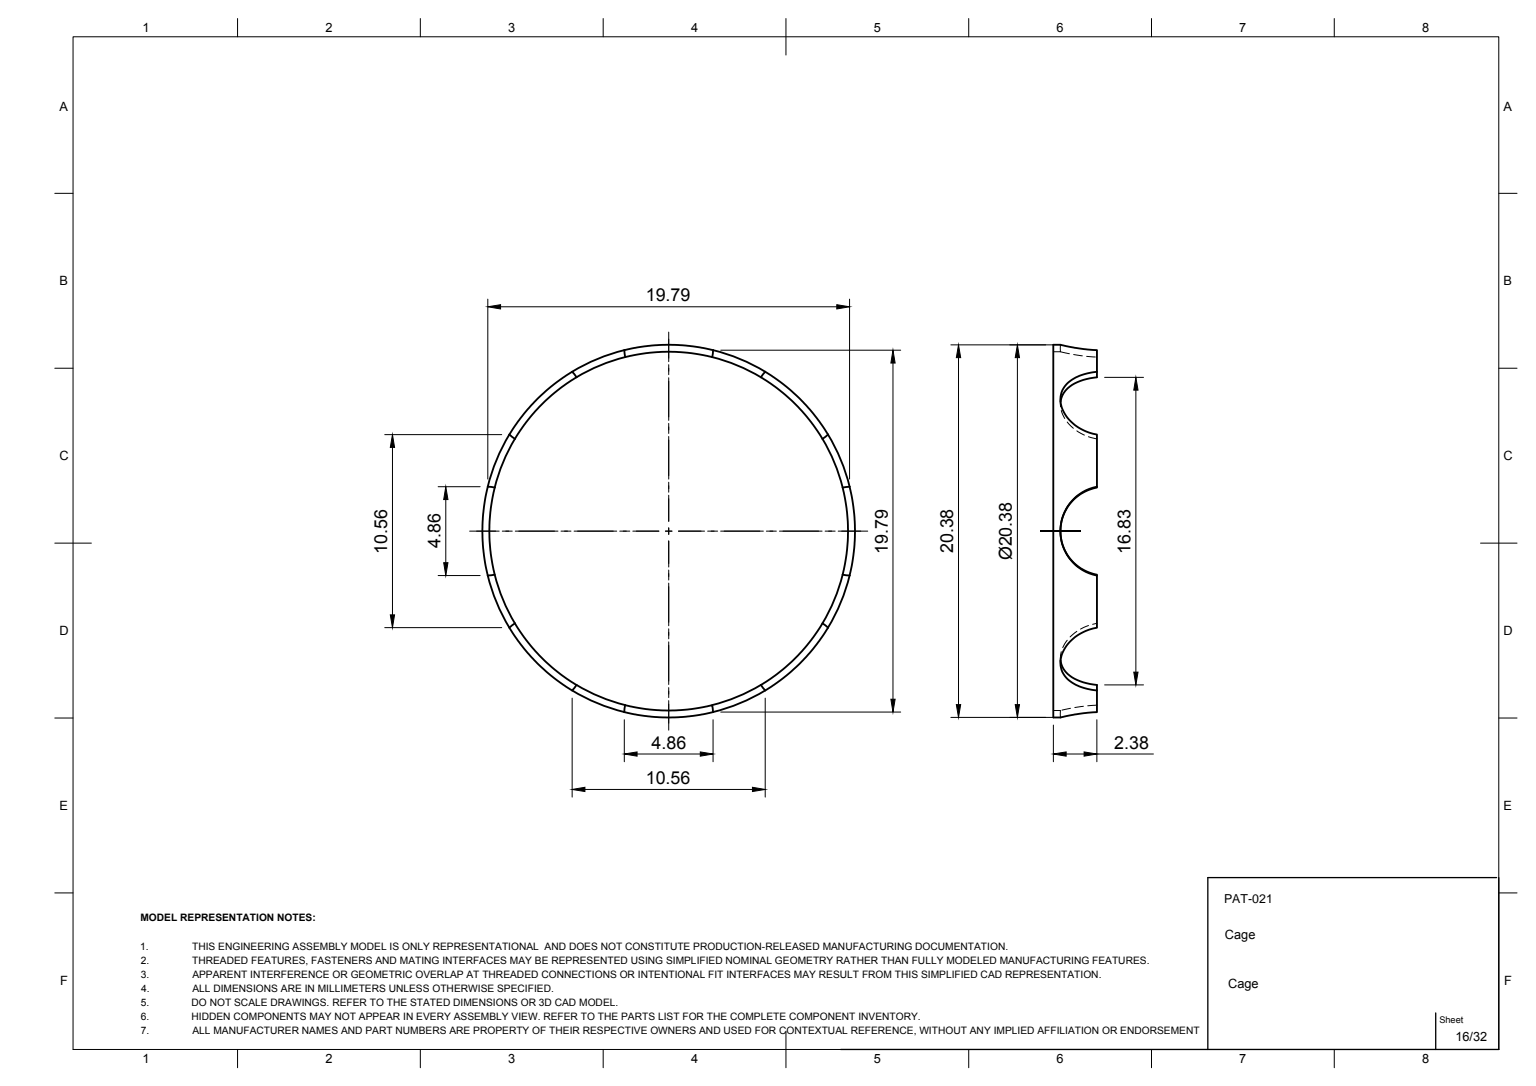
ISO-10303-21;
HEADER;
/* Generated by software containing ST-Developer
 * from STEP Tools, Inc. (www.steptools.com) 
 */

FILE_DESCRIPTION(
/* description */ ('Chain-less indexing wheel (Geneva) drive'),
/* implementation_level */ '2;1');

FILE_NAME(
/* name */ 'Cage.step',
/* time_stamp */ '2026-10-28T03:25:22-07:00',
/* author */ (''),
/* organization */ (''),
/* preprocessor_version */ 'ST-DEVELOPER v20.2',
/* originating_system */ 'Autodesk Translation Framework v15.17.0.0',
/* authorisation */ '');

FILE_SCHEMA (('AUTOMOTIVE_DESIGN { 1 0 10303 214 3 1 1 }'));
ENDSEC;

DATA;
#10=MECHANICAL_DESIGN_GEOMETRIC_PRESENTATION_REPRESENTATION('',(#320),#10957);
#187=SPHERICAL_SURFACE('',#6329,0.247676);
#188=SPHERICAL_SURFACE('',#6345,0.247676);
#189=SPHERICAL_SURFACE('',#6350,0.247676);
#190=SPHERICAL_SURFACE('',#6355,0.247676);
#191=SPHERICAL_SURFACE('',#6360,0.247676);
#192=SPHERICAL_SURFACE('',#6365,0.247676);
#193=SPHERICAL_SURFACE('',#6370,0.247676);
#194=SPHERICAL_SURFACE('',#6378,0.247676);
#215=B_SPLINE_CURVE_WITH_KNOTS('',3,(#9357,#9358,#9359,#9360,#9361,#9362,
#9363,#9364,#9365,#9366,#9367,#9368,#9369,#9370,#9371,#9372,#9373,#9374,
#9375,#9376,#9377,#9378),.UNSPECIFIED.,.F.,.F.,(4,2,2,2,2,2,2,2,2,2,4),
(0.0473477652366656,0.126350602536658,0.189525903804987,0.252701205073317,
0.313298422430275,0.373895639787233,0.434492857144191,0.495090074501149,
0.558265375769478,0.621440677037807,0.7004435143378),.UNSPECIFIED.);
#216=B_SPLINE_CURVE_WITH_KNOTS('',3,(#9382,#9383,#9384,#9385,#9386,#9387,
#9388,#9389,#9390,#9391,#9392,#9393,#9394,#9395,#9396,#9397,#9398,#9399,
#9400,#9401,#9402,#9403),.UNSPECIFIED.,.F.,.F.,(4,2,2,2,2,2,2,2,2,2,4),
(0.0464897534940957,0.0852567806515119,0.170513561303024,0.246687263103517,
0.308657850341199,0.370628437578881,0.432599024816563,0.494569612054245,
0.570743313854739,0.656000094506251,0.694767121663666),.UNSPECIFIED.);
#217=B_SPLINE_CURVE_WITH_KNOTS('',3,(#9409,#9410,#9411,#9412,#9413,#9414,
#9415,#9416,#9417,#9418,#9419,#9420,#9421,#9422,#9423,#9424,#9425,#9426,
#9427,#9428,#9429,#9430),.UNSPECIFIED.,.F.,.F.,(4,2,2,2,2,2,2,2,2,2,4),
(0.0464897534940957,0.0852567806515118,0.170513561303024,0.246687263103517,
0.308657850341199,0.370628437578881,0.432599024816563,0.494569612054245,
0.570743313854738,0.65600009450625,0.694767121663666),.UNSPECIFIED.);
#218=B_SPLINE_CURVE_WITH_KNOTS('',3,(#9434,#9435,#9436,#9437,#9438,#9439,
#9440,#9441,#9442,#9443,#9444,#9445,#9446,#9447,#9448,#9449,#9450,#9451,
#9452,#9453,#9454,#9455),.UNSPECIFIED.,.F.,.F.,(4,2,2,2,2,2,2,2,2,2,4),
(0.0464897534940957,0.0852567806515119,0.170513561303024,0.246687263103517,
0.308657850341199,0.370628437578881,0.432599024816563,0.494569612054245,
0.570743313854739,0.656000094506251,0.694767121663666),.UNSPECIFIED.);
#219=B_SPLINE_CURVE_WITH_KNOTS('',3,(#9459,#9460,#9461,#9462,#9463,#9464,
#9465,#9466,#9467,#9468,#9469,#9470),.UNSPECIFIED.,.F.,.F.,(4,2,2,2,2,4),
(0.0464897534940957,0.0852567806515119,0.170513561303024,0.246687263103517,
0.308657850341199,0.370628437578881),.UNSPECIFIED.);
#220=B_SPLINE_CURVE_WITH_KNOTS('',3,(#9475,#9476,#9477,#9478,#9479,#9480,
#9481,#9482,#9483,#9484,#9485,#9486),.UNSPECIFIED.,.F.,.F.,(4,2,2,2,2,4),
(0.370628437578881,0.432599024816563,0.494569612054245,0.570743313854738,
0.65600009450625,0.694767121663666),.UNSPECIFIED.);
#221=B_SPLINE_CURVE_WITH_KNOTS('',3,(#9490,#9491,#9492,#9493,#9494,#9495,
#9496,#9497,#9498,#9499,#9500,#9501,#9502,#9503,#9504,#9505,#9506,#9507,
#9508,#9509,#9510,#9511),.UNSPECIFIED.,.F.,.F.,(4,2,2,2,2,2,2,2,2,2,4),
(0.0464897534940957,0.0852567806515121,0.170513561303024,0.246687263103518,
0.308657850341199,0.370628437578881,0.432599024816563,0.494569612054245,
0.570743313854738,0.65600009450625,0.694767121663666),.UNSPECIFIED.);
#222=B_SPLINE_CURVE_WITH_KNOTS('',3,(#9515,#9516,#9517,#9518,#9519,#9520,
#9521,#9522,#9523,#9524,#9525,#9526,#9527,#9528,#9529,#9530,#9531,#9532,
#9533,#9534,#9535,#9536),.UNSPECIFIED.,.F.,.F.,(4,2,2,2,2,2,2,2,2,2,4),
(0.0464897534940957,0.0852567806515119,0.170513561303024,0.246687263103517,
0.308657850341199,0.370628437578881,0.432599024816563,0.494569612054245,
0.570743313854738,0.65600009450625,0.694767121663667),.UNSPECIFIED.);
#223=B_SPLINE_CURVE_WITH_KNOTS('',3,(#9540,#9541,#9542,#9543,#9544,#9545,
#9546,#9547,#9548,#9549,#9550,#9551,#9552,#9553,#9554,#9555,#9556,#9557,
#9558,#9559,#9560,#9561),.UNSPECIFIED.,.F.,.F.,(4,2,2,2,2,2,2,2,2,2,4),
(0.0464897534940957,0.0852567806515119,0.170513561303024,0.246687263103517,
0.308657850341199,0.370628437578881,0.432599024816563,0.494569612054245,
0.570743313854738,0.65600009450625,0.694767121663666),.UNSPECIFIED.);
#224=B_SPLINE_CURVE_WITH_KNOTS('',3,(#9565,#9566,#9567,#9568,#9569,#9570,
#9571,#9572,#9573,#9574,#9575,#9576,#9577,#9578,#9579,#9580,#9581,#9582,
#9583,#9584,#9585,#9586),.UNSPECIFIED.,.F.,.F.,(4,2,2,2,2,2,2,2,2,2,4),
(0.0464897534940957,0.0852567806515119,0.170513561303024,0.246687263103517,
0.308657850341199,0.370628437578881,0.432599024816563,0.494569612054245,
0.570743313854739,0.656000094506251,0.694767121663667),.UNSPECIFIED.);
#225=B_SPLINE_CURVE_WITH_KNOTS('',3,(#9594,#9595,#9596,#9597,#9598,#9599,
#9600,#9601,#9602,#9603,#9604,#9605,#9606,#9607,#9608,#9609,#9610,#9611,
#9612,#9613,#9614,#9615),.UNSPECIFIED.,.F.,.F.,(4,2,2,2,2,2,2,2,2,2,4),
(0.0473477652366656,0.126350602536658,0.189525903804987,0.252701205073316,
0.313298422430274,0.373895639787232,0.434492857144191,0.495090074501149,
0.558265375769478,0.621440677037807,0.7004435143378),.UNSPECIFIED.);
#226=B_SPLINE_CURVE_WITH_KNOTS('',3,(#9623,#9624,#9625,#9626,#9627,#9628,
#9629,#9630,#9631,#9632,#9633,#9634,#9635,#9636,#9637,#9638,#9639,#9640,
#9641,#9642,#9643,#9644),.UNSPECIFIED.,.F.,.F.,(4,2,2,2,2,2,2,2,2,2,4),
(0.0473477652366656,0.126350602536658,0.189525903804987,0.252701205073317,
0.313298422430275,0.373895639787233,0.434492857144191,0.495090074501149,
0.558265375769478,0.621440677037807,0.7004435143378),.UNSPECIFIED.);
#227=B_SPLINE_CURVE_WITH_KNOTS('',3,(#9653,#9654,#9655,#9656,#9657,#9658,
#9659,#9660,#9661,#9662,#9663,#9664),.UNSPECIFIED.,.F.,.F.,(4,2,2,2,2,4),
(0.0473477652366656,0.126350602536658,0.189525903804987,0.252701205073316,
0.313298422430275,0.373895639787233),.UNSPECIFIED.);
#228=B_SPLINE_CURVE_WITH_KNOTS('',3,(#9666,#9667,#9668,#9669,#9670,#9671,
#9672,#9673,#9674,#9675,#9676,#9677),.UNSPECIFIED.,.F.,.F.,(4,2,2,2,2,4),
(0.373895639787233,0.434492857144191,0.495090074501149,0.558265375769478,
0.621440677037807,0.7004435143378),.UNSPECIFIED.);
#229=B_SPLINE_CURVE_WITH_KNOTS('',3,(#9684,#9685,#9686,#9687,#9688,#9689,
#9690,#9691,#9692,#9693,#9694,#9695,#9696,#9697,#9698,#9699,#9700,#9701,
#9702,#9703,#9704,#9705),.UNSPECIFIED.,.F.,.F.,(4,2,2,2,2,2,2,2,2,2,4),
(0.0473477652366656,0.126350602536658,0.189525903804987,0.252701205073316,
0.313298422430275,0.373895639787233,0.434492857144191,0.495090074501149,
0.558265375769478,0.621440677037807,0.7004435143378),.UNSPECIFIED.);
#230=B_SPLINE_CURVE_WITH_KNOTS('',3,(#9713,#9714,#9715,#9716,#9717,#9718,
#9719,#9720,#9721,#9722,#9723,#9724,#9725,#9726,#9727,#9728,#9729,#9730,
#9731,#9732,#9733,#9734),.UNSPECIFIED.,.F.,.F.,(4,2,2,2,2,2,2,2,2,2,4),
(0.0473477652366656,0.126350602536658,0.189525903804987,0.252701205073317,
0.313298422430275,0.373895639787233,0.434492857144191,0.495090074501149,
0.558265375769478,0.621440677037807,0.7004435143378),.UNSPECIFIED.);
#231=B_SPLINE_CURVE_WITH_KNOTS('',3,(#9742,#9743,#9744,#9745,#9746,#9747,
#9748,#9749,#9750,#9751,#9752,#9753,#9754,#9755,#9756,#9757,#9758,#9759,
#9760,#9761,#9762,#9763),.UNSPECIFIED.,.F.,.F.,(4,2,2,2,2,2,2,2,2,2,4),
(0.0473477652366656,0.126350602536658,0.189525903804987,0.252701205073316,
0.313298422430275,0.373895639787233,0.434492857144191,0.495090074501149,
0.558265375769478,0.621440677037807,0.7004435143378),.UNSPECIFIED.);
#232=B_SPLINE_CURVE_WITH_KNOTS('',3,(#9772,#9773,#9774,#9775,#9776,#9777,
#9778,#9779,#9780,#9781,#9782,#9783,#9784,#9785,#9786,#9787,#9788,#9789,
#9790,#9791,#9792,#9793),.UNSPECIFIED.,.F.,.F.,(4,2,2,2,2,2,2,2,2,2,4),
(0.0473477652366656,0.126350602536658,0.189525903804987,0.252701205073317,
0.313298422430275,0.373895639787233,0.434492857144191,0.495090074501149,
0.558265375769478,0.621440677037807,0.7004435143378),.UNSPECIFIED.);
#263=SHAPE_REPRESENTATION_RELATIONSHIP('SRR','None',#11077,#288);
#288=ADVANCED_BREP_SHAPE_REPRESENTATION('',(#352),#10940);
#320=STYLED_ITEM('',(#11287),#352);
#352=MANIFOLD_SOLID_BREP('Continuous crown cage',#5717);
#428=FACE_BOUND('',#1213,.T.);
#543=PLANE('',#6342);
#544=PLANE('',#6347);
#545=PLANE('',#6352);
#546=PLANE('',#6357);
#547=PLANE('',#6362);
#548=PLANE('',#6367);
#549=PLANE('',#6376);
#550=PLANE('',#6380);
#551=PLANE('',#6381);
#801=FACE_OUTER_BOUND('',#1195,.T.);
#802=FACE_OUTER_BOUND('',#1196,.T.);
#803=FACE_OUTER_BOUND('',#1197,.T.);
#804=FACE_OUTER_BOUND('',#1198,.T.);
#805=FACE_OUTER_BOUND('',#1199,.T.);
#806=FACE_OUTER_BOUND('',#1200,.T.);
#807=FACE_OUTER_BOUND('',#1201,.T.);
#808=FACE_OUTER_BOUND('',#1202,.T.);
#809=FACE_OUTER_BOUND('',#1203,.T.);
#810=FACE_OUTER_BOUND('',#1204,.T.);
#811=FACE_OUTER_BOUND('',#1205,.T.);
#812=FACE_OUTER_BOUND('',#1206,.T.);
#813=FACE_OUTER_BOUND('',#1207,.T.);
#814=FACE_OUTER_BOUND('',#1208,.T.);
#815=FACE_OUTER_BOUND('',#1209,.T.);
#816=FACE_OUTER_BOUND('',#1210,.T.);
#817=FACE_OUTER_BOUND('',#1211,.T.);
#818=FACE_OUTER_BOUND('',#1212,.T.);
#819=FACE_OUTER_BOUND('',#1214,.T.);
#1195=EDGE_LOOP('',(#4379,#4380,#4381,#4382));
#1196=EDGE_LOOP('',(#4383,#4384,#4385,#4386,#4387,#4388,#4389,#4390,#4391,
#4392,#4393,#4394,#4395,#4396,#4397,#4398,#4399,#4400,#4401,#4402));
#1197=EDGE_LOOP('',(#4403,#4404,#4405,#4406));
#1198=EDGE_LOOP('',(#4407,#4408,#4409,#4410));
#1199=EDGE_LOOP('',(#4411,#4412,#4413,#4414));
#1200=EDGE_LOOP('',(#4415,#4416,#4417,#4418));
#1201=EDGE_LOOP('',(#4419,#4420,#4421,#4422));
#1202=EDGE_LOOP('',(#4423,#4424,#4425,#4426,#4427,#4428));
#1203=EDGE_LOOP('',(#4429,#4430,#4431,#4432));
#1204=EDGE_LOOP('',(#4433,#4434,#4435,#4436));
#1205=EDGE_LOOP('',(#4437,#4438,#4439,#4440));
#1206=EDGE_LOOP('',(#4441,#4442,#4443,#4444));
#1207=EDGE_LOOP('',(#4445,#4446,#4447,#4448));
#1208=EDGE_LOOP('',(#4449,#4450,#4451,#4452));
#1209=EDGE_LOOP('',(#4453,#4454,#4455,#4456,#4457,#4458,#4459,#4460,#4461,
#4462,#4463,#4464,#4465,#4466,#4467,#4468,#4469,#4470,#4471,#4472));
#1210=EDGE_LOOP('',(#4473,#4474,#4475,#4476));
#1211=EDGE_LOOP('',(#4477,#4478,#4479,#4480));
#1212=EDGE_LOOP('',(#4481));
#1213=EDGE_LOOP('',(#4482));
#1214=EDGE_LOOP('',(#4483,#4484,#4485,#4486));
#1581=LINE('',#9472,#1955);
#1582=LINE('',#9768,#1956);
#1955=VECTOR('',#7559,1.019052);
#1956=VECTOR('',#7636,0.980948);
#2327=CIRCLE('',#6330,0.243053047864041);
#2328=CIRCLE('',#6331,0.243053047864041);
#2329=CIRCLE('',#6333,1.019052);
#2330=CIRCLE('',#6334,1.019052);
#2331=CIRCLE('',#6335,1.019052);
#2332=CIRCLE('',#6336,1.019052);
#2333=CIRCLE('',#6337,1.019052);
#2334=CIRCLE('',#6338,1.019052);
#2335=CIRCLE('',#6339,1.019052);
#2336=CIRCLE('',#6340,1.019052);
#2337=CIRCLE('',#6341,1.019052);
#2338=CIRCLE('',#6343,0.980948);
#2339=CIRCLE('',#6344,0.243053047864041);
#2340=CIRCLE('',#6346,0.243053047864041);
#2341=CIRCLE('',#6348,0.980948);
#2342=CIRCLE('',#6349,0.243053047864041);
#2343=CIRCLE('',#6351,0.243053047864041);
#2344=CIRCLE('',#6353,0.980948);
#2345=CIRCLE('',#6354,0.243053047864041);
#2346=CIRCLE('',#6356,0.243053047864041);
#2347=CIRCLE('',#6358,0.980948);
#2348=CIRCLE('',#6359,0.243053047864041);
#2349=CIRCLE('',#6361,0.243053047864041);
#2350=CIRCLE('',#6363,0.980948);
#2351=CIRCLE('',#6364,0.243053047864041);
#2352=CIRCLE('',#6366,0.243053047864041);
#2353=CIRCLE('',#6368,0.980948);
#2354=CIRCLE('',#6369,0.243053047864041);
#2355=CIRCLE('',#6371,0.243053047864041);
#2356=CIRCLE('',#6373,0.980948);
#2357=CIRCLE('',#6374,0.980948);
#2358=CIRCLE('',#6375,0.980948);
#2359=CIRCLE('',#6377,0.243053047864041);
#2360=CIRCLE('',#6379,0.243053047864041);
#2713=VERTEX_POINT('',#9355);
#2714=VERTEX_POINT('',#9356);
#2715=VERTEX_POINT('',#9379);
#2716=VERTEX_POINT('',#9381);
#2717=VERTEX_POINT('',#9406);
#2718=VERTEX_POINT('',#9408);
#2719=VERTEX_POINT('',#9431);
#2720=VERTEX_POINT('',#9433);
#2721=VERTEX_POINT('',#9456);
#2722=VERTEX_POINT('',#9458);
#2723=VERTEX_POINT('',#9471);
#2724=VERTEX_POINT('',#9474);
#2725=VERTEX_POINT('',#9487);
#2726=VERTEX_POINT('',#9489);
#2727=VERTEX_POINT('',#9512);
#2728=VERTEX_POINT('',#9514);
#2729=VERTEX_POINT('',#9537);
#2730=VERTEX_POINT('',#9539);
#2731=VERTEX_POINT('',#9562);
#2732=VERTEX_POINT('',#9564);
#2733=VERTEX_POINT('',#9589);
#2734=VERTEX_POINT('',#9593);
#2735=VERTEX_POINT('',#9618);
#2736=VERTEX_POINT('',#9622);
#2737=VERTEX_POINT('',#9647);
#2738=VERTEX_POINT('',#9651);
#2739=VERTEX_POINT('',#9652);
#2740=VERTEX_POINT('',#9679);
#2741=VERTEX_POINT('',#9683);
#2742=VERTEX_POINT('',#9708);
#2743=VERTEX_POINT('',#9712);
#2744=VERTEX_POINT('',#9737);
#2745=VERTEX_POINT('',#9741);
#2746=VERTEX_POINT('',#9766);
#2747=VERTEX_POINT('',#9769);
#2748=VERTEX_POINT('',#9771);
#3315=EDGE_CURVE('',#2713,#2714,#215,.T.);
#3316=EDGE_CURVE('',#2715,#2713,#2327,.T.);
#3317=EDGE_CURVE('',#2716,#2715,#216,.T.);
#3318=EDGE_CURVE('',#2714,#2716,#2328,.T.);
#3319=EDGE_CURVE('',#2717,#2715,#2329,.T.);
#3320=EDGE_CURVE('',#2717,#2718,#217,.T.);
#3321=EDGE_CURVE('',#2719,#2718,#2330,.T.);
#3322=EDGE_CURVE('',#2719,#2720,#218,.T.);
#3323=EDGE_CURVE('',#2721,#2720,#2331,.T.);
#3324=EDGE_CURVE('',#2721,#2722,#219,.T.);
#3325=EDGE_CURVE('',#2722,#2723,#1581,.T.);
#3326=EDGE_CURVE('',#2723,#2723,#2332,.T.);
#3327=EDGE_CURVE('',#2722,#2724,#220,.T.);
#3328=EDGE_CURVE('',#2725,#2724,#2333,.T.);
#3329=EDGE_CURVE('',#2725,#2726,#221,.T.);
#3330=EDGE_CURVE('',#2727,#2726,#2334,.T.);
#3331=EDGE_CURVE('',#2727,#2728,#222,.T.);
#3332=EDGE_CURVE('',#2729,#2728,#2335,.T.);
#3333=EDGE_CURVE('',#2729,#2730,#223,.T.);
#3334=EDGE_CURVE('',#2731,#2730,#2336,.T.);
#3335=EDGE_CURVE('',#2731,#2732,#224,.T.);
#3336=EDGE_CURVE('',#2716,#2732,#2337,.T.);
#3337=EDGE_CURVE('',#2713,#2733,#2338,.T.);
#3338=EDGE_CURVE('',#2733,#2717,#2339,.T.);
#3339=EDGE_CURVE('',#2734,#2733,#225,.T.);
#3340=EDGE_CURVE('',#2718,#2734,#2340,.T.);
#3341=EDGE_CURVE('',#2734,#2735,#2341,.T.);
#3342=EDGE_CURVE('',#2735,#2719,#2342,.T.);
#3343=EDGE_CURVE('',#2736,#2735,#226,.T.);
#3344=EDGE_CURVE('',#2720,#2736,#2343,.T.);
#3345=EDGE_CURVE('',#2736,#2737,#2344,.T.);
#3346=EDGE_CURVE('',#2737,#2721,#2345,.T.);
#3347=EDGE_CURVE('',#2738,#2739,#227,.T.);
#3348=EDGE_CURVE('',#2724,#2738,#2346,.T.);
#3349=EDGE_CURVE('',#2739,#2737,#228,.T.);
#3350=EDGE_CURVE('',#2738,#2740,#2347,.T.);
#3351=EDGE_CURVE('',#2740,#2725,#2348,.T.);
#3352=EDGE_CURVE('',#2741,#2740,#229,.T.);
#3353=EDGE_CURVE('',#2726,#2741,#2349,.T.);
#3354=EDGE_CURVE('',#2741,#2742,#2350,.T.);
#3355=EDGE_CURVE('',#2742,#2727,#2351,.T.);
#3356=EDGE_CURVE('',#2743,#2742,#230,.T.);
#3357=EDGE_CURVE('',#2728,#2743,#2352,.T.);
#3358=EDGE_CURVE('',#2743,#2744,#2353,.T.);
#3359=EDGE_CURVE('',#2744,#2729,#2354,.T.);
#3360=EDGE_CURVE('',#2745,#2744,#231,.T.);
#3361=EDGE_CURVE('',#2730,#2745,#2355,.T.);
#3362=EDGE_CURVE('',#2746,#2746,#2356,.T.);
#3363=EDGE_CURVE('',#2746,#2739,#1582,.T.);
#3364=EDGE_CURVE('',#2747,#2714,#2357,.T.);
#3365=EDGE_CURVE('',#2747,#2748,#232,.T.);
#3366=EDGE_CURVE('',#2745,#2748,#2358,.T.);
#3367=EDGE_CURVE('',#2732,#2747,#2359,.T.);
#3368=EDGE_CURVE('',#2748,#2731,#2360,.T.);
#4379=ORIENTED_EDGE('',*,*,#3315,.F.);
#4380=ORIENTED_EDGE('',*,*,#3316,.F.);
#4381=ORIENTED_EDGE('',*,*,#3317,.F.);
#4382=ORIENTED_EDGE('',*,*,#3318,.F.);
#4383=ORIENTED_EDGE('',*,*,#3317,.T.);
#4384=ORIENTED_EDGE('',*,*,#3319,.F.);
#4385=ORIENTED_EDGE('',*,*,#3320,.T.);
#4386=ORIENTED_EDGE('',*,*,#3321,.F.);
#4387=ORIENTED_EDGE('',*,*,#3322,.T.);
#4388=ORIENTED_EDGE('',*,*,#3323,.F.);
#4389=ORIENTED_EDGE('',*,*,#3324,.T.);
#4390=ORIENTED_EDGE('',*,*,#3325,.T.);
#4391=ORIENTED_EDGE('',*,*,#3326,.F.);
#4392=ORIENTED_EDGE('',*,*,#3325,.F.);
#4393=ORIENTED_EDGE('',*,*,#3327,.T.);
#4394=ORIENTED_EDGE('',*,*,#3328,.F.);
#4395=ORIENTED_EDGE('',*,*,#3329,.T.);
#4396=ORIENTED_EDGE('',*,*,#3330,.F.);
#4397=ORIENTED_EDGE('',*,*,#3331,.T.);
#4398=ORIENTED_EDGE('',*,*,#3332,.F.);
#4399=ORIENTED_EDGE('',*,*,#3333,.T.);
#4400=ORIENTED_EDGE('',*,*,#3334,.F.);
#4401=ORIENTED_EDGE('',*,*,#3335,.T.);
#4402=ORIENTED_EDGE('',*,*,#3336,.F.);
#4403=ORIENTED_EDGE('',*,*,#3316,.T.);
#4404=ORIENTED_EDGE('',*,*,#3337,.T.);
#4405=ORIENTED_EDGE('',*,*,#3338,.T.);
#4406=ORIENTED_EDGE('',*,*,#3319,.T.);
#4407=ORIENTED_EDGE('',*,*,#3339,.F.);
#4408=ORIENTED_EDGE('',*,*,#3340,.F.);
#4409=ORIENTED_EDGE('',*,*,#3320,.F.);
#4410=ORIENTED_EDGE('',*,*,#3338,.F.);
#4411=ORIENTED_EDGE('',*,*,#3340,.T.);
#4412=ORIENTED_EDGE('',*,*,#3341,.T.);
#4413=ORIENTED_EDGE('',*,*,#3342,.T.);
#4414=ORIENTED_EDGE('',*,*,#3321,.T.);
#4415=ORIENTED_EDGE('',*,*,#3343,.F.);
#4416=ORIENTED_EDGE('',*,*,#3344,.F.);
#4417=ORIENTED_EDGE('',*,*,#3322,.F.);
#4418=ORIENTED_EDGE('',*,*,#3342,.F.);
#4419=ORIENTED_EDGE('',*,*,#3344,.T.);
#4420=ORIENTED_EDGE('',*,*,#3345,.T.);
#4421=ORIENTED_EDGE('',*,*,#3346,.T.);
#4422=ORIENTED_EDGE('',*,*,#3323,.T.);
#4423=ORIENTED_EDGE('',*,*,#3347,.F.);
#4424=ORIENTED_EDGE('',*,*,#3348,.F.);
#4425=ORIENTED_EDGE('',*,*,#3327,.F.);
#4426=ORIENTED_EDGE('',*,*,#3324,.F.);
#4427=ORIENTED_EDGE('',*,*,#3346,.F.);
#4428=ORIENTED_EDGE('',*,*,#3349,.F.);
#4429=ORIENTED_EDGE('',*,*,#3348,.T.);
#4430=ORIENTED_EDGE('',*,*,#3350,.T.);
#4431=ORIENTED_EDGE('',*,*,#3351,.T.);
#4432=ORIENTED_EDGE('',*,*,#3328,.T.);
#4433=ORIENTED_EDGE('',*,*,#3352,.F.);
#4434=ORIENTED_EDGE('',*,*,#3353,.F.);
#4435=ORIENTED_EDGE('',*,*,#3329,.F.);
#4436=ORIENTED_EDGE('',*,*,#3351,.F.);
#4437=ORIENTED_EDGE('',*,*,#3353,.T.);
#4438=ORIENTED_EDGE('',*,*,#3354,.T.);
#4439=ORIENTED_EDGE('',*,*,#3355,.T.);
#4440=ORIENTED_EDGE('',*,*,#3330,.T.);
#4441=ORIENTED_EDGE('',*,*,#3356,.F.);
#4442=ORIENTED_EDGE('',*,*,#3357,.F.);
#4443=ORIENTED_EDGE('',*,*,#3331,.F.);
#4444=ORIENTED_EDGE('',*,*,#3355,.F.);
#4445=ORIENTED_EDGE('',*,*,#3357,.T.);
#4446=ORIENTED_EDGE('',*,*,#3358,.T.);
#4447=ORIENTED_EDGE('',*,*,#3359,.T.);
#4448=ORIENTED_EDGE('',*,*,#3332,.T.);
#4449=ORIENTED_EDGE('',*,*,#3333,.F.);
#4450=ORIENTED_EDGE('',*,*,#3359,.F.);
#4451=ORIENTED_EDGE('',*,*,#3360,.F.);
#4452=ORIENTED_EDGE('',*,*,#3361,.F.);
#4453=ORIENTED_EDGE('',*,*,#3362,.F.);
#4454=ORIENTED_EDGE('',*,*,#3363,.T.);
#4455=ORIENTED_EDGE('',*,*,#3349,.T.);
#4456=ORIENTED_EDGE('',*,*,#3345,.F.);
#4457=ORIENTED_EDGE('',*,*,#3343,.T.);
#4458=ORIENTED_EDGE('',*,*,#3341,.F.);
#4459=ORIENTED_EDGE('',*,*,#3339,.T.);
#4460=ORIENTED_EDGE('',*,*,#3337,.F.);
#4461=ORIENTED_EDGE('',*,*,#3315,.T.);
#4462=ORIENTED_EDGE('',*,*,#3364,.F.);
#4463=ORIENTED_EDGE('',*,*,#3365,.T.);
#4464=ORIENTED_EDGE('',*,*,#3366,.F.);
#4465=ORIENTED_EDGE('',*,*,#3360,.T.);
#4466=ORIENTED_EDGE('',*,*,#3358,.F.);
#4467=ORIENTED_EDGE('',*,*,#3356,.T.);
#4468=ORIENTED_EDGE('',*,*,#3354,.F.);
#4469=ORIENTED_EDGE('',*,*,#3352,.T.);
#4470=ORIENTED_EDGE('',*,*,#3350,.F.);
#4471=ORIENTED_EDGE('',*,*,#3347,.T.);
#4472=ORIENTED_EDGE('',*,*,#3363,.F.);
#4473=ORIENTED_EDGE('',*,*,#3318,.T.);
#4474=ORIENTED_EDGE('',*,*,#3336,.T.);
#4475=ORIENTED_EDGE('',*,*,#3367,.T.);
#4476=ORIENTED_EDGE('',*,*,#3364,.T.);
#4477=ORIENTED_EDGE('',*,*,#3335,.F.);
#4478=ORIENTED_EDGE('',*,*,#3368,.F.);
#4479=ORIENTED_EDGE('',*,*,#3365,.F.);
#4480=ORIENTED_EDGE('',*,*,#3367,.F.);
#4481=ORIENTED_EDGE('',*,*,#3326,.T.);
#4482=ORIENTED_EDGE('',*,*,#3362,.T.);
#4483=ORIENTED_EDGE('',*,*,#3361,.T.);
#4484=ORIENTED_EDGE('',*,*,#3366,.T.);
#4485=ORIENTED_EDGE('',*,*,#3368,.T.);
#4486=ORIENTED_EDGE('',*,*,#3334,.T.);
#5303=CYLINDRICAL_SURFACE('',#6332,1.019052);
#5304=CYLINDRICAL_SURFACE('',#6372,0.980948);
#5515=ADVANCED_FACE('',(#801),#187,.F.);
#5516=ADVANCED_FACE('',(#802),#5303,.T.);
#5517=ADVANCED_FACE('',(#803),#543,.T.);
#5518=ADVANCED_FACE('',(#804),#188,.F.);
#5519=ADVANCED_FACE('',(#805),#544,.T.);
#5520=ADVANCED_FACE('',(#806),#189,.F.);
#5521=ADVANCED_FACE('',(#807),#545,.T.);
#5522=ADVANCED_FACE('',(#808),#190,.F.);
#5523=ADVANCED_FACE('',(#809),#546,.T.);
#5524=ADVANCED_FACE('',(#810),#191,.F.);
#5525=ADVANCED_FACE('',(#811),#547,.T.);
#5526=ADVANCED_FACE('',(#812),#192,.F.);
#5527=ADVANCED_FACE('',(#813),#548,.T.);
#5528=ADVANCED_FACE('',(#814),#193,.F.);
#5529=ADVANCED_FACE('',(#815),#5304,.F.);
#5530=ADVANCED_FACE('',(#816),#549,.T.);
#5531=ADVANCED_FACE('',(#817),#194,.F.);
#5532=ADVANCED_FACE('',(#818,#428),#550,.T.);
#5533=ADVANCED_FACE('',(#819),#551,.T.);
#5717=CLOSED_SHELL('',(#5515,#5516,#5517,#5518,#5519,#5520,#5521,#5522,
#5523,#5524,#5525,#5526,#5527,#5528,#5529,#5530,#5531,#5532,#5533));
#6328=AXIS2_PLACEMENT_3D('',#9353,#7543,#7544);
#6329=AXIS2_PLACEMENT_3D('',#9354,#7545,#7546);
#6330=AXIS2_PLACEMENT_3D('',#9380,#7547,#7548);
#6331=AXIS2_PLACEMENT_3D('',#9404,#7549,#7550);
#6332=AXIS2_PLACEMENT_3D('',#9405,#7551,#7552);
#6333=AXIS2_PLACEMENT_3D('',#9407,#7553,#7554);
#6334=AXIS2_PLACEMENT_3D('',#9432,#7555,#7556);
#6335=AXIS2_PLACEMENT_3D('',#9457,#7557,#7558);
#6336=AXIS2_PLACEMENT_3D('',#9473,#7560,#7561);
#6337=AXIS2_PLACEMENT_3D('',#9488,#7562,#7563);
#6338=AXIS2_PLACEMENT_3D('',#9513,#7564,#7565);
#6339=AXIS2_PLACEMENT_3D('',#9538,#7566,#7567);
#6340=AXIS2_PLACEMENT_3D('',#9563,#7568,#7569);
#6341=AXIS2_PLACEMENT_3D('',#9587,#7570,#7571);
#6342=AXIS2_PLACEMENT_3D('',#9588,#7572,#7573);
#6343=AXIS2_PLACEMENT_3D('',#9590,#7574,#7575);
#6344=AXIS2_PLACEMENT_3D('',#9591,#7576,#7577);
#6345=AXIS2_PLACEMENT_3D('',#9592,#7578,#7579);
#6346=AXIS2_PLACEMENT_3D('',#9616,#7580,#7581);
#6347=AXIS2_PLACEMENT_3D('',#9617,#7582,#7583);
#6348=AXIS2_PLACEMENT_3D('',#9619,#7584,#7585);
#6349=AXIS2_PLACEMENT_3D('',#9620,#7586,#7587);
#6350=AXIS2_PLACEMENT_3D('',#9621,#7588,#7589);
#6351=AXIS2_PLACEMENT_3D('',#9645,#7590,#7591);
#6352=AXIS2_PLACEMENT_3D('',#9646,#7592,#7593);
#6353=AXIS2_PLACEMENT_3D('',#9648,#7594,#7595);
#6354=AXIS2_PLACEMENT_3D('',#9649,#7596,#7597);
#6355=AXIS2_PLACEMENT_3D('',#9650,#7598,#7599);
#6356=AXIS2_PLACEMENT_3D('',#9665,#7600,#7601);
#6357=AXIS2_PLACEMENT_3D('',#9678,#7602,#7603);
#6358=AXIS2_PLACEMENT_3D('',#9680,#7604,#7605);
#6359=AXIS2_PLACEMENT_3D('',#9681,#7606,#7607);
#6360=AXIS2_PLACEMENT_3D('',#9682,#7608,#7609);
#6361=AXIS2_PLACEMENT_3D('',#9706,#7610,#7611);
#6362=AXIS2_PLACEMENT_3D('',#9707,#7612,#7613);
#6363=AXIS2_PLACEMENT_3D('',#9709,#7614,#7615);
#6364=AXIS2_PLACEMENT_3D('',#9710,#7616,#7617);
#6365=AXIS2_PLACEMENT_3D('',#9711,#7618,#7619);
#6366=AXIS2_PLACEMENT_3D('',#9735,#7620,#7621);
#6367=AXIS2_PLACEMENT_3D('',#9736,#7622,#7623);
#6368=AXIS2_PLACEMENT_3D('',#9738,#7624,#7625);
#6369=AXIS2_PLACEMENT_3D('',#9739,#7626,#7627);
#6370=AXIS2_PLACEMENT_3D('',#9740,#7628,#7629);
#6371=AXIS2_PLACEMENT_3D('',#9764,#7630,#7631);
#6372=AXIS2_PLACEMENT_3D('',#9765,#7632,#7633);
#6373=AXIS2_PLACEMENT_3D('',#9767,#7634,#7635);
#6374=AXIS2_PLACEMENT_3D('',#9770,#7637,#7638);
#6375=AXIS2_PLACEMENT_3D('',#9794,#7639,#7640);
#6376=AXIS2_PLACEMENT_3D('',#9795,#7641,#7642);
#6377=AXIS2_PLACEMENT_3D('',#9796,#7643,#7644);
#6378=AXIS2_PLACEMENT_3D('',#9797,#7645,#7646);
#6379=AXIS2_PLACEMENT_3D('',#9798,#7647,#7648);
#6380=AXIS2_PLACEMENT_3D('',#9799,#7649,#7650);
#6381=AXIS2_PLACEMENT_3D('',#9800,#7651,#7652);
#7543=DIRECTION('axis',(0.,0.,1.));
#7544=DIRECTION('refdir',(1.,0.,0.));
#7545=DIRECTION('center_axis',(0.,0.,1.));
#7546=DIRECTION('ref_axis',(1.,0.,0.));
#7547=DIRECTION('center_axis',(0.,-1.,0.));
#7548=DIRECTION('ref_axis',(0.,0.,-1.));
#7549=DIRECTION('center_axis',(0.,-1.,0.));
#7550=DIRECTION('ref_axis',(0.,0.,-1.));
#7551=DIRECTION('center_axis',(0.,1.,0.));
#7552=DIRECTION('ref_axis',(1.,0.,0.));
#7553=DIRECTION('center_axis',(0.,1.,0.));
#7554=DIRECTION('ref_axis',(1.,0.,0.));
#7555=DIRECTION('center_axis',(0.,1.,0.));
#7556=DIRECTION('ref_axis',(1.,0.,0.));
#7557=DIRECTION('center_axis',(0.,1.,0.));
#7558=DIRECTION('ref_axis',(1.,0.,0.));
#7559=DIRECTION('',(0.,-1.,0.));
#7560=DIRECTION('center_axis',(0.,-1.,0.));
#7561=DIRECTION('ref_axis',(1.,0.,0.));
#7562=DIRECTION('center_axis',(0.,1.,0.));
#7563=DIRECTION('ref_axis',(1.,0.,0.));
#7564=DIRECTION('center_axis',(0.,1.,0.));
#7565=DIRECTION('ref_axis',(1.,0.,0.));
#7566=DIRECTION('center_axis',(0.,1.,0.));
#7567=DIRECTION('ref_axis',(1.,0.,0.));
#7568=DIRECTION('center_axis',(0.,1.,0.));
#7569=DIRECTION('ref_axis',(1.,0.,0.));
#7570=DIRECTION('center_axis',(0.,1.,0.));
#7571=DIRECTION('ref_axis',(1.,0.,0.));
#7572=DIRECTION('center_axis',(0.,1.,0.));
#7573=DIRECTION('ref_axis',(1.,0.,0.));
#7574=DIRECTION('center_axis',(0.,-1.,0.));
#7575=DIRECTION('ref_axis',(1.,0.,0.));
#7576=DIRECTION('center_axis',(0.,-1.,0.));
#7577=DIRECTION('ref_axis',(0.,0.,-1.));
#7578=DIRECTION('center_axis',(6.12323399573677E-17,0.,1.));
#7579=DIRECTION('ref_axis',(1.,0.,0.));
#7580=DIRECTION('center_axis',(0.,-1.,0.));
#7581=DIRECTION('ref_axis',(0.,0.,-1.));
#7582=DIRECTION('center_axis',(0.,1.,0.));
#7583=DIRECTION('ref_axis',(1.,0.,0.));
#7584=DIRECTION('center_axis',(0.,-1.,0.));
#7585=DIRECTION('ref_axis',(1.,0.,0.));
#7586=DIRECTION('center_axis',(0.,-1.,0.));
#7587=DIRECTION('ref_axis',(0.,0.,-1.));
#7588=DIRECTION('center_axis',(0.,0.,1.));
#7589=DIRECTION('ref_axis',(1.,0.,0.));
#7590=DIRECTION('center_axis',(0.,-1.,0.));
#7591=DIRECTION('ref_axis',(0.,0.,-1.));
#7592=DIRECTION('center_axis',(0.,1.,0.));
#7593=DIRECTION('ref_axis',(1.,0.,0.));
#7594=DIRECTION('center_axis',(0.,-1.,0.));
#7595=DIRECTION('ref_axis',(1.,0.,0.));
#7596=DIRECTION('center_axis',(0.,-1.,0.));
#7597=DIRECTION('ref_axis',(0.,0.,-1.));
#7598=DIRECTION('center_axis',(0.,0.,1.));
#7599=DIRECTION('ref_axis',(1.,0.,0.));
#7600=DIRECTION('center_axis',(0.,-1.,0.));
#7601=DIRECTION('ref_axis',(0.,0.,-1.));
#7602=DIRECTION('center_axis',(0.,1.,0.));
#7603=DIRECTION('ref_axis',(1.,0.,0.));
#7604=DIRECTION('center_axis',(0.,-1.,0.));
#7605=DIRECTION('ref_axis',(1.,0.,0.));
#7606=DIRECTION('center_axis',(0.,-1.,0.));
#7607=DIRECTION('ref_axis',(0.,0.,-1.));
#7608=DIRECTION('center_axis',(0.,0.,1.));
#7609=DIRECTION('ref_axis',(1.,0.,0.));
#7610=DIRECTION('center_axis',(0.,-1.,0.));
#7611=DIRECTION('ref_axis',(0.,0.,-1.));
#7612=DIRECTION('center_axis',(0.,1.,0.));
#7613=DIRECTION('ref_axis',(1.,0.,0.));
#7614=DIRECTION('center_axis',(0.,-1.,0.));
#7615=DIRECTION('ref_axis',(1.,0.,0.));
#7616=DIRECTION('center_axis',(0.,-1.,0.));
#7617=DIRECTION('ref_axis',(0.,0.,-1.));
#7618=DIRECTION('center_axis',(6.12323399573676E-17,0.,1.));
#7619=DIRECTION('ref_axis',(1.,0.,0.));
#7620=DIRECTION('center_axis',(0.,-1.,0.));
#7621=DIRECTION('ref_axis',(0.,0.,-1.));
#7622=DIRECTION('center_axis',(0.,1.,0.));
#7623=DIRECTION('ref_axis',(1.,0.,0.));
#7624=DIRECTION('center_axis',(0.,-1.,0.));
#7625=DIRECTION('ref_axis',(1.,0.,0.));
#7626=DIRECTION('center_axis',(0.,-1.,0.));
#7627=DIRECTION('ref_axis',(0.,0.,-1.));
#7628=DIRECTION('center_axis',(0.,0.,1.));
#7629=DIRECTION('ref_axis',(1.,0.,0.));
#7630=DIRECTION('center_axis',(0.,-1.,0.));
#7631=DIRECTION('ref_axis',(0.,0.,-1.));
#7632=DIRECTION('center_axis',(0.,1.,0.));
#7633=DIRECTION('ref_axis',(1.,0.,0.));
#7634=DIRECTION('center_axis',(0.,1.,0.));
#7635=DIRECTION('ref_axis',(1.,0.,0.));
#7636=DIRECTION('',(0.,1.,0.));
#7637=DIRECTION('center_axis',(0.,-1.,0.));
#7638=DIRECTION('ref_axis',(1.,0.,0.));
#7639=DIRECTION('center_axis',(0.,-1.,0.));
#7640=DIRECTION('ref_axis',(1.,0.,0.));
#7641=DIRECTION('center_axis',(0.,1.,0.));
#7642=DIRECTION('ref_axis',(1.,0.,0.));
#7643=DIRECTION('center_axis',(0.,-1.,0.));
#7644=DIRECTION('ref_axis',(0.,0.,-1.));
#7645=DIRECTION('center_axis',(0.,0.,1.));
#7646=DIRECTION('ref_axis',(1.,0.,0.));
#7647=DIRECTION('center_axis',(0.,-1.,0.));
#7648=DIRECTION('ref_axis',(0.,0.,-1.));
#7649=DIRECTION('center_axis',(0.,-1.,0.));
#7650=DIRECTION('ref_axis',(-1.,0.,0.));
#7651=DIRECTION('center_axis',(0.,1.,0.));
#7652=DIRECTION('ref_axis',(1.,0.,0.));
#9353=CARTESIAN_POINT('',(0.,0.,0.));
#9354=CARTESIAN_POINT('Origin',(0.707106781186547,0.,0.707106781186548));
#9355=CARTESIAN_POINT('',(0.504455939115715,-0.04763,0.841298510752802));
#9356=CARTESIAN_POINT('',(0.841298510752802,-0.04763,0.504455939115715));
#9357=CARTESIAN_POINT('Ctrl Pts',(0.504455939115715,-0.04763,0.841298510752802));
#9358=CARTESIAN_POINT('Ctrl Pts',(0.508899795931835,-0.0740444353928835,
0.838633903678357));
#9359=CARTESIAN_POINT('Ctrl Pts',(0.517157748491652,-0.0999305678883309,
0.833661031856294));
#9360=CARTESIAN_POINT('Ctrl Pts',(0.537715343527944,-0.142345102874864,
0.820511285096538));
#9361=CARTESIAN_POINT('Ctrl Pts',(0.548874290046456,-0.159766064500479,
0.813159949759));
#9362=CARTESIAN_POINT('Ctrl Pts',(0.573915184558107,-0.190326085855194,
0.795684265985089));
#9363=CARTESIAN_POINT('Ctrl Pts',(0.587792702767295,-0.203463743702801,
0.78555112003688));
#9364=CARTESIAN_POINT('Ctrl Pts',(0.615966552324775,-0.224161999508995,
0.763642258217233));
#9365=CARTESIAN_POINT('Ctrl Pts',(0.631684198665438,-0.232861760990032,
0.750785745543687));
#9366=CARTESIAN_POINT('Ctrl Pts',(0.663382628119203,-0.244251601209411,
0.722929908501543));
#9367=CARTESIAN_POINT('Ctrl Pts',(0.679352081686668,-0.246942143572133,
0.707917883896095));
#9368=CARTESIAN_POINT('Ctrl Pts',(0.707917883896095,-0.246942143572133,
0.679352081686668));
#9369=CARTESIAN_POINT('Ctrl Pts',(0.722929908501543,-0.244251601209411,
0.663382628119203));
#9370=CARTESIAN_POINT('Ctrl Pts',(0.750785745543687,-0.232861760990032,
0.631684198665439));
#9371=CARTESIAN_POINT('Ctrl Pts',(0.763642258217232,-0.224161999508995,
0.615966552324775));
#9372=CARTESIAN_POINT('Ctrl Pts',(0.78555112003688,-0.203463743702801,0.587792702767295));
#9373=CARTESIAN_POINT('Ctrl Pts',(0.795684265985088,-0.190326085855194,
0.573915184558108));
#9374=CARTESIAN_POINT('Ctrl Pts',(0.813159949759,-0.15976606450048,0.548874290046456));
#9375=CARTESIAN_POINT('Ctrl Pts',(0.820511285096538,-0.142345102874864,
0.537715343527944));
#9376=CARTESIAN_POINT('Ctrl Pts',(0.833661031856294,-0.099930567888331,
0.517157748491653));
#9377=CARTESIAN_POINT('Ctrl Pts',(0.838633903678357,-0.0740444353928835,
0.508899795931835));
#9378=CARTESIAN_POINT('Ctrl Pts',(0.841298510752801,-0.0476299999999999,
0.504455939115715));
#9379=CARTESIAN_POINT('',(0.528110872004958,-0.04763,0.871530771444223));
#9380=CARTESIAN_POINT('Origin',(0.707106781186547,-0.04763,0.707106781186548));
#9381=CARTESIAN_POINT('',(0.871530771444223,-0.04763,0.528110872004959));
#9382=CARTESIAN_POINT('Ctrl Pts',(0.871530771444223,-0.0476300000000001,
0.528110872004958));
#9383=CARTESIAN_POINT('Ctrl Pts',(0.87014664509073,-0.0609922781173483,
0.530395067942936));
#9384=CARTESIAN_POINT('Ctrl Pts',(0.868149331745851,-0.0742967091364493,
0.533674141594226));
#9385=CARTESIAN_POINT('Ctrl Pts',(0.85981294420286,-0.115492077056649,0.54708917182331));
#9386=CARTESIAN_POINT('Ctrl Pts',(0.850993704737257,-0.141695629206859,
0.560922177770136));
#9387=CARTESIAN_POINT('Ctrl Pts',(0.830754510485543,-0.181890537957859,
0.590422647829571));
#9388=CARTESIAN_POINT('Ctrl Pts',(0.816896541396381,-0.201072148666545,
0.609616703125488));
#9389=CARTESIAN_POINT('Ctrl Pts',(0.792310597819928,-0.223955109275652,
0.641117951819998));
#9390=CARTESIAN_POINT('Ctrl Pts',(0.779109323683612,-0.232742381310829,
0.657208095763053));
#9391=CARTESIAN_POINT('Ctrl Pts',(0.750552691816206,-0.244234834628584,
0.68964083160521));
#9392=CARTESIAN_POINT('Ctrl Pts',(0.735185187071673,-0.246942143572133,
0.705971972091755));
#9393=CARTESIAN_POINT('Ctrl Pts',(0.705971972091754,-0.246942143572133,
0.735185187071673));
#9394=CARTESIAN_POINT('Ctrl Pts',(0.689640831605209,-0.244234834628584,
0.750552691816206));
#9395=CARTESIAN_POINT('Ctrl Pts',(0.657208095763052,-0.232742381310829,
0.779109323683612));
#9396=CARTESIAN_POINT('Ctrl Pts',(0.641117951819998,-0.223955109275652,
0.792310597819928));
#9397=CARTESIAN_POINT('Ctrl Pts',(0.609616703125487,-0.201072148666545,
0.816896541396382));
#9398=CARTESIAN_POINT('Ctrl Pts',(0.590422647829571,-0.181890537957858,
0.830754510485544));
#9399=CARTESIAN_POINT('Ctrl Pts',(0.560922177770135,-0.141695629206858,
0.850993704737257));
#9400=CARTESIAN_POINT('Ctrl Pts',(0.547089171823309,-0.115492077056649,
0.859812944202861));
#9401=CARTESIAN_POINT('Ctrl Pts',(0.533674141594226,-0.0742967091364491,
0.868149331745852));
#9402=CARTESIAN_POINT('Ctrl Pts',(0.530395067942936,-0.0609922781173483,
0.870146645090731));
#9403=CARTESIAN_POINT('Ctrl Pts',(0.528110872004958,-0.0476300000000001,
0.871530771444223));
#9404=CARTESIAN_POINT('Origin',(0.707106781186547,-0.04763,0.707106781186548));
#9405=CARTESIAN_POINT('Origin',(0.,-0.166705,0.));
#9406=CARTESIAN_POINT('',(0.242834539687906,-0.04763,0.989696097314));
#9407=CARTESIAN_POINT('Origin',(0.,-0.04763,0.));
#9408=CARTESIAN_POINT('',(-0.242834539687907,-0.04763,0.989696097314));
#9409=CARTESIAN_POINT('Ctrl Pts',(0.242834539687906,-0.04763,0.989696097314));
#9410=CARTESIAN_POINT('Ctrl Pts',(0.24024064412003,-0.0609922781173483,
0.990332542620729));
#9411=CARTESIAN_POINT('Ctrl Pts',(0.236509675094874,-0.0742967091364492,
0.991238884025248));
#9412=CARTESIAN_POINT('Ctrl Pts',(0.221129100087819,-0.115492077056649,
0.994830026707808));
#9413=CARTESIAN_POINT('Ctrl Pts',(0.205111543747588,-0.141695629206859,
0.998375294985966));
#9414=CARTESIAN_POINT('Ctrl Pts',(0.169940289819232,-0.181890537957859,
1.00492400591205));
#9415=CARTESIAN_POINT('Ctrl Pts',(0.1465689792446,-0.201072148666545,1.00869718865384));
#9416=CARTESIAN_POINT('Ctrl Pts',(0.106909345252087,-0.223955109275652,
1.01358704779679));
#9417=CARTESIAN_POINT('Ctrl Pts',(0.0861971848975941,-0.232742381310829,
1.0156297872271));
#9418=CARTESIAN_POINT('Ctrl Pts',(0.0430711894098822,-0.244234834628584,
1.01837060663223));
#9419=CARTESIAN_POINT('Ctrl Pts',(0.0206568624125605,-0.246942143572133,
1.019052));
#9420=CARTESIAN_POINT('Ctrl Pts',(-0.0206568624125608,-0.246942143572133,
1.019052));
#9421=CARTESIAN_POINT('Ctrl Pts',(-0.0430711894098825,-0.244234834628584,
1.01837060663223));
#9422=CARTESIAN_POINT('Ctrl Pts',(-0.0861971848975943,-0.232742381310829,
1.0156297872271));
#9423=CARTESIAN_POINT('Ctrl Pts',(-0.106909345252088,-0.223955109275652,
1.01358704779679));
#9424=CARTESIAN_POINT('Ctrl Pts',(-0.1465689792446,-0.201072148666545,1.00869718865384));
#9425=CARTESIAN_POINT('Ctrl Pts',(-0.169940289819232,-0.181890537957859,
1.00492400591205));
#9426=CARTESIAN_POINT('Ctrl Pts',(-0.205111543747588,-0.141695629206859,
0.998375294985966));
#9427=CARTESIAN_POINT('Ctrl Pts',(-0.221129100087819,-0.115492077056649,
0.994830026707808));
#9428=CARTESIAN_POINT('Ctrl Pts',(-0.236509675094875,-0.0742967091364493,
0.991238884025248));
#9429=CARTESIAN_POINT('Ctrl Pts',(-0.24024064412003,-0.0609922781173483,
0.990332542620729));
#9430=CARTESIAN_POINT('Ctrl Pts',(-0.242834539687907,-0.04763,0.989696097314));
#9431=CARTESIAN_POINT('',(-0.528110872004959,-0.04763,0.871530771444223));
#9432=CARTESIAN_POINT('Origin',(0.,-0.04763,0.));
#9433=CARTESIAN_POINT('',(-0.871530771444223,-0.04763,0.528110872004958));
#9434=CARTESIAN_POINT('Ctrl Pts',(-0.528110872004958,-0.0476300000000001,
0.871530771444223));
#9435=CARTESIAN_POINT('Ctrl Pts',(-0.530395067942936,-0.0609922781173484,
0.87014664509073));
#9436=CARTESIAN_POINT('Ctrl Pts',(-0.533674141594226,-0.0742967091364493,
0.868149331745851));
#9437=CARTESIAN_POINT('Ctrl Pts',(-0.54708917182331,-0.115492077056649,
0.85981294420286));
#9438=CARTESIAN_POINT('Ctrl Pts',(-0.560922177770136,-0.141695629206859,
0.850993704737257));
#9439=CARTESIAN_POINT('Ctrl Pts',(-0.590422647829571,-0.181890537957859,
0.830754510485543));
#9440=CARTESIAN_POINT('Ctrl Pts',(-0.609616703125488,-0.201072148666545,
0.816896541396381));
#9441=CARTESIAN_POINT('Ctrl Pts',(-0.641117951819998,-0.223955109275652,
0.792310597819928));
#9442=CARTESIAN_POINT('Ctrl Pts',(-0.657208095763053,-0.232742381310829,
0.779109323683611));
#9443=CARTESIAN_POINT('Ctrl Pts',(-0.68964083160521,-0.244234834628584,
0.750552691816205));
#9444=CARTESIAN_POINT('Ctrl Pts',(-0.705971972091755,-0.246942143572133,
0.735185187071673));
#9445=CARTESIAN_POINT('Ctrl Pts',(-0.735185187071673,-0.246942143572133,
0.705971972091754));
#9446=CARTESIAN_POINT('Ctrl Pts',(-0.750552691816206,-0.244234834628584,
0.689640831605209));
#9447=CARTESIAN_POINT('Ctrl Pts',(-0.779109323683612,-0.232742381310829,
0.657208095763052));
#9448=CARTESIAN_POINT('Ctrl Pts',(-0.792310597819928,-0.223955109275652,
0.641117951819998));
#9449=CARTESIAN_POINT('Ctrl Pts',(-0.816896541396382,-0.201072148666545,
0.609616703125487));
#9450=CARTESIAN_POINT('Ctrl Pts',(-0.830754510485544,-0.181890537957858,
0.590422647829571));
#9451=CARTESIAN_POINT('Ctrl Pts',(-0.850993704737257,-0.141695629206858,
0.560922177770135));
#9452=CARTESIAN_POINT('Ctrl Pts',(-0.859812944202861,-0.115492077056649,
0.547089171823309));
#9453=CARTESIAN_POINT('Ctrl Pts',(-0.868149331745852,-0.0742967091364491,
0.533674141594226));
#9454=CARTESIAN_POINT('Ctrl Pts',(-0.870146645090731,-0.0609922781173483,
0.530395067942936));
#9455=CARTESIAN_POINT('Ctrl Pts',(-0.871530771444223,-0.04763,0.528110872004958));
#9456=CARTESIAN_POINT('',(-0.989696097314,-0.04763,0.242834539687906));
#9457=CARTESIAN_POINT('Origin',(0.,-0.04763,0.));
#9458=CARTESIAN_POINT('',(-1.019052,-0.246942143572133,1.248489836334E-16));
#9459=CARTESIAN_POINT('Ctrl Pts',(-0.989696097314,-0.04763,0.242834539687906));
#9460=CARTESIAN_POINT('Ctrl Pts',(-0.990332542620729,-0.0609922781173483,
0.24024064412003));
#9461=CARTESIAN_POINT('Ctrl Pts',(-0.991238884025248,-0.0742967091364492,
0.236509675094874));
#9462=CARTESIAN_POINT('Ctrl Pts',(-0.994830026707808,-0.115492077056649,
0.221129100087819));
#9463=CARTESIAN_POINT('Ctrl Pts',(-0.998375294985966,-0.141695629206859,
0.205111543747588));
#9464=CARTESIAN_POINT('Ctrl Pts',(-1.00492400591205,-0.181890537957859,
0.169940289819232));
#9465=CARTESIAN_POINT('Ctrl Pts',(-1.00869718865384,-0.201072148666545,
0.1465689792446));
#9466=CARTESIAN_POINT('Ctrl Pts',(-1.01358704779679,-0.223955109275652,
0.106909345252088));
#9467=CARTESIAN_POINT('Ctrl Pts',(-1.0156297872271,-0.232742381310829,0.0861971848975944));
#9468=CARTESIAN_POINT('Ctrl Pts',(-1.01837060663223,-0.244234834628584,
0.0430711894098825));
#9469=CARTESIAN_POINT('Ctrl Pts',(-1.019052,-0.246942143572133,0.0206568624125608));
#9470=CARTESIAN_POINT('Ctrl Pts',(-1.019052,-0.246942143572133,1.2490009027033E-16));
#9471=CARTESIAN_POINT('',(-1.019052,-0.28578,1.24797876996471E-16));
#9472=CARTESIAN_POINT('',(-1.019052,-0.166705,1.24797876996471E-16));
#9473=CARTESIAN_POINT('Origin',(0.,-0.28578,0.));
#9474=CARTESIAN_POINT('',(-0.989696097314,-0.04763,-0.242834539687906));
#9475=CARTESIAN_POINT('Ctrl Pts',(-1.019052,-0.246942143572133,1.2490009027033E-16));
#9476=CARTESIAN_POINT('Ctrl Pts',(-1.019052,-0.246942143572133,-0.0206568624125605));
#9477=CARTESIAN_POINT('Ctrl Pts',(-1.01837060663223,-0.244234834628584,
-0.0430711894098822));
#9478=CARTESIAN_POINT('Ctrl Pts',(-1.0156297872271,-0.232742381310829,-0.0861971848975941));
#9479=CARTESIAN_POINT('Ctrl Pts',(-1.01358704779679,-0.223955109275652,
-0.106909345252087));
#9480=CARTESIAN_POINT('Ctrl Pts',(-1.00869718865384,-0.201072148666546,
-0.1465689792446));
#9481=CARTESIAN_POINT('Ctrl Pts',(-1.00492400591205,-0.181890537957859,
-0.169940289819232));
#9482=CARTESIAN_POINT('Ctrl Pts',(-0.998375294985966,-0.141695629206859,
-0.205111543747588));
#9483=CARTESIAN_POINT('Ctrl Pts',(-0.994830026707808,-0.11549207705665,
-0.221129100087819));
#9484=CARTESIAN_POINT('Ctrl Pts',(-0.991238884025248,-0.0742967091364495,
-0.236509675094874));
#9485=CARTESIAN_POINT('Ctrl Pts',(-0.990332542620729,-0.0609922781173484,
-0.24024064412003));
#9486=CARTESIAN_POINT('Ctrl Pts',(-0.989696097314,-0.0476300000000001,-0.242834539687907));
#9487=CARTESIAN_POINT('',(-0.871530771444223,-0.04763,-0.528110872004958));
#9488=CARTESIAN_POINT('Origin',(0.,-0.04763,0.));
#9489=CARTESIAN_POINT('',(-0.528110872004958,-0.04763,-0.871530771444223));
#9490=CARTESIAN_POINT('Ctrl Pts',(-0.871530771444223,-0.0476300000000001,
-0.528110872004958));
#9491=CARTESIAN_POINT('Ctrl Pts',(-0.87014664509073,-0.0609922781173484,
-0.530395067942936));
#9492=CARTESIAN_POINT('Ctrl Pts',(-0.868149331745851,-0.0742967091364494,
-0.533674141594226));
#9493=CARTESIAN_POINT('Ctrl Pts',(-0.85981294420286,-0.115492077056649,
-0.54708917182331));
#9494=CARTESIAN_POINT('Ctrl Pts',(-0.850993704737257,-0.141695629206859,
-0.560922177770136));
#9495=CARTESIAN_POINT('Ctrl Pts',(-0.830754510485543,-0.181890537957859,
-0.590422647829571));
#9496=CARTESIAN_POINT('Ctrl Pts',(-0.816896541396381,-0.201072148666546,
-0.609616703125488));
#9497=CARTESIAN_POINT('Ctrl Pts',(-0.792310597819928,-0.223955109275652,
-0.641117951819999));
#9498=CARTESIAN_POINT('Ctrl Pts',(-0.779109323683611,-0.232742381310829,
-0.657208095763053));
#9499=CARTESIAN_POINT('Ctrl Pts',(-0.750552691816205,-0.244234834628584,
-0.68964083160521));
#9500=CARTESIAN_POINT('Ctrl Pts',(-0.735185187071673,-0.246942143572133,
-0.705971972091755));
#9501=CARTESIAN_POINT('Ctrl Pts',(-0.705971972091754,-0.246942143572133,
-0.735185187071673));
#9502=CARTESIAN_POINT('Ctrl Pts',(-0.68964083160521,-0.244234834628584,
-0.750552691816206));
#9503=CARTESIAN_POINT('Ctrl Pts',(-0.657208095763052,-0.232742381310829,
-0.779109323683612));
#9504=CARTESIAN_POINT('Ctrl Pts',(-0.641117951819998,-0.223955109275652,
-0.792310597819928));
#9505=CARTESIAN_POINT('Ctrl Pts',(-0.609616703125488,-0.201072148666545,
-0.816896541396381));
#9506=CARTESIAN_POINT('Ctrl Pts',(-0.590422647829571,-0.181890537957859,
-0.830754510485543));
#9507=CARTESIAN_POINT('Ctrl Pts',(-0.560922177770136,-0.141695629206859,
-0.850993704737257));
#9508=CARTESIAN_POINT('Ctrl Pts',(-0.54708917182331,-0.115492077056649,
-0.85981294420286));
#9509=CARTESIAN_POINT('Ctrl Pts',(-0.533674141594226,-0.0742967091364494,
-0.868149331745852));
#9510=CARTESIAN_POINT('Ctrl Pts',(-0.530395067942936,-0.0609922781173484,
-0.870146645090731));
#9511=CARTESIAN_POINT('Ctrl Pts',(-0.528110872004958,-0.0476300000000001,
-0.871530771444223));
#9512=CARTESIAN_POINT('',(-0.242834539687906,-0.04763,-0.989696097314));
#9513=CARTESIAN_POINT('Origin',(0.,-0.04763,0.));
#9514=CARTESIAN_POINT('',(0.242834539687906,-0.04763,-0.989696097314));
#9515=CARTESIAN_POINT('Ctrl Pts',(-0.242834539687907,-0.04763,-0.989696097314));
#9516=CARTESIAN_POINT('Ctrl Pts',(-0.24024064412003,-0.0609922781173483,
-0.990332542620729));
#9517=CARTESIAN_POINT('Ctrl Pts',(-0.236509675094874,-0.0742967091364493,
-0.991238884025248));
#9518=CARTESIAN_POINT('Ctrl Pts',(-0.221129100087819,-0.115492077056649,
-0.994830026707808));
#9519=CARTESIAN_POINT('Ctrl Pts',(-0.205111543747588,-0.141695629206859,
-0.998375294985966));
#9520=CARTESIAN_POINT('Ctrl Pts',(-0.169940289819232,-0.181890537957859,
-1.00492400591205));
#9521=CARTESIAN_POINT('Ctrl Pts',(-0.1465689792446,-0.201072148666545,-1.00869718865384));
#9522=CARTESIAN_POINT('Ctrl Pts',(-0.106909345252087,-0.223955109275652,
-1.01358704779679));
#9523=CARTESIAN_POINT('Ctrl Pts',(-0.0861971848975942,-0.232742381310829,
-1.0156297872271));
#9524=CARTESIAN_POINT('Ctrl Pts',(-0.0430711894098823,-0.244234834628584,
-1.01837060663223));
#9525=CARTESIAN_POINT('Ctrl Pts',(-0.0206568624125606,-0.246942143572133,
-1.019052));
#9526=CARTESIAN_POINT('Ctrl Pts',(0.0206568624125607,-0.246942143572133,
-1.019052));
#9527=CARTESIAN_POINT('Ctrl Pts',(0.0430711894098824,-0.244234834628584,
-1.01837060663223));
#9528=CARTESIAN_POINT('Ctrl Pts',(0.0861971848975943,-0.232742381310829,
-1.0156297872271));
#9529=CARTESIAN_POINT('Ctrl Pts',(0.106909345252088,-0.223955109275652,
-1.01358704779679));
#9530=CARTESIAN_POINT('Ctrl Pts',(0.1465689792446,-0.201072148666545,-1.00869718865384));
#9531=CARTESIAN_POINT('Ctrl Pts',(0.169940289819232,-0.181890537957859,
-1.00492400591205));
#9532=CARTESIAN_POINT('Ctrl Pts',(0.205111543747588,-0.141695629206859,
-0.998375294985966));
#9533=CARTESIAN_POINT('Ctrl Pts',(0.221129100087819,-0.115492077056649,
-0.994830026707808));
#9534=CARTESIAN_POINT('Ctrl Pts',(0.236509675094874,-0.0742967091364493,
-0.991238884025248));
#9535=CARTESIAN_POINT('Ctrl Pts',(0.24024064412003,-0.0609922781173484,
-0.990332542620729));
#9536=CARTESIAN_POINT('Ctrl Pts',(0.242834539687907,-0.04763,-0.989696097314));
#9537=CARTESIAN_POINT('',(0.528110872004958,-0.04763,-0.871530771444223));
#9538=CARTESIAN_POINT('Origin',(0.,-0.04763,0.));
#9539=CARTESIAN_POINT('',(0.871530771444223,-0.04763,-0.528110872004958));
#9540=CARTESIAN_POINT('Ctrl Pts',(0.528110872004958,-0.0476300000000001,
-0.871530771444223));
#9541=CARTESIAN_POINT('Ctrl Pts',(0.530395067942936,-0.0609922781173484,
-0.870146645090731));
#9542=CARTESIAN_POINT('Ctrl Pts',(0.533674141594226,-0.0742967091364493,
-0.868149331745851));
#9543=CARTESIAN_POINT('Ctrl Pts',(0.54708917182331,-0.115492077056649,-0.85981294420286));
#9544=CARTESIAN_POINT('Ctrl Pts',(0.560922177770136,-0.141695629206859,
-0.850993704737257));
#9545=CARTESIAN_POINT('Ctrl Pts',(0.590422647829571,-0.181890537957859,
-0.830754510485543));
#9546=CARTESIAN_POINT('Ctrl Pts',(0.609616703125488,-0.201072148666545,
-0.816896541396381));
#9547=CARTESIAN_POINT('Ctrl Pts',(0.641117951819998,-0.223955109275652,
-0.792310597819928));
#9548=CARTESIAN_POINT('Ctrl Pts',(0.657208095763053,-0.232742381310829,
-0.779109323683612));
#9549=CARTESIAN_POINT('Ctrl Pts',(0.68964083160521,-0.244234834628584,-0.750552691816206));
#9550=CARTESIAN_POINT('Ctrl Pts',(0.705971972091755,-0.246942143572133,
-0.735185187071673));
#9551=CARTESIAN_POINT('Ctrl Pts',(0.735185187071673,-0.246942143572133,
-0.705971972091754));
#9552=CARTESIAN_POINT('Ctrl Pts',(0.750552691816206,-0.244234834628584,
-0.68964083160521));
#9553=CARTESIAN_POINT('Ctrl Pts',(0.779109323683612,-0.232742381310829,
-0.657208095763053));
#9554=CARTESIAN_POINT('Ctrl Pts',(0.792310597819928,-0.223955109275652,
-0.641117951819998));
#9555=CARTESIAN_POINT('Ctrl Pts',(0.816896541396381,-0.201072148666545,
-0.609616703125488));
#9556=CARTESIAN_POINT('Ctrl Pts',(0.830754510485543,-0.181890537957859,
-0.590422647829571));
#9557=CARTESIAN_POINT('Ctrl Pts',(0.850993704737257,-0.141695629206859,
-0.560922177770136));
#9558=CARTESIAN_POINT('Ctrl Pts',(0.85981294420286,-0.115492077056649,-0.54708917182331));
#9559=CARTESIAN_POINT('Ctrl Pts',(0.868149331745851,-0.0742967091364493,
-0.533674141594226));
#9560=CARTESIAN_POINT('Ctrl Pts',(0.870146645090731,-0.0609922781173484,
-0.530395067942936));
#9561=CARTESIAN_POINT('Ctrl Pts',(0.871530771444223,-0.0476300000000001,
-0.528110872004958));
#9562=CARTESIAN_POINT('',(0.989696097314,-0.04763,-0.242834539687906));
#9563=CARTESIAN_POINT('Origin',(0.,-0.04763,0.));
#9564=CARTESIAN_POINT('',(0.989696097314,-0.04763,0.242834539687906));
#9565=CARTESIAN_POINT('Ctrl Pts',(0.989696097314,-0.04763,-0.242834539687907));
#9566=CARTESIAN_POINT('Ctrl Pts',(0.990332542620729,-0.0609922781173483,
-0.24024064412003));
#9567=CARTESIAN_POINT('Ctrl Pts',(0.991238884025248,-0.0742967091364493,
-0.236509675094874));
#9568=CARTESIAN_POINT('Ctrl Pts',(0.994830026707808,-0.115492077056649,
-0.221129100087819));
#9569=CARTESIAN_POINT('Ctrl Pts',(0.998375294985966,-0.141695629206859,
-0.205111543747588));
#9570=CARTESIAN_POINT('Ctrl Pts',(1.00492400591205,-0.181890537957859,-0.169940289819232));
#9571=CARTESIAN_POINT('Ctrl Pts',(1.00869718865384,-0.201072148666545,-0.1465689792446));
#9572=CARTESIAN_POINT('Ctrl Pts',(1.01358704779679,-0.223955109275652,-0.106909345252087));
#9573=CARTESIAN_POINT('Ctrl Pts',(1.0156297872271,-0.232742381310829,-0.0861971848975942));
#9574=CARTESIAN_POINT('Ctrl Pts',(1.01837060663223,-0.244234834628584,-0.0430711894098823));
#9575=CARTESIAN_POINT('Ctrl Pts',(1.019052,-0.246942143572133,-0.0206568624125607));
#9576=CARTESIAN_POINT('Ctrl Pts',(1.019052,-0.246942143572133,0.0206568624125607));
#9577=CARTESIAN_POINT('Ctrl Pts',(1.01837060663223,-0.244234834628584,0.0430711894098823));
#9578=CARTESIAN_POINT('Ctrl Pts',(1.0156297872271,-0.232742381310829,0.0861971848975942));
#9579=CARTESIAN_POINT('Ctrl Pts',(1.01358704779679,-0.223955109275652,0.106909345252087));
#9580=CARTESIAN_POINT('Ctrl Pts',(1.00869718865384,-0.201072148666545,0.1465689792446));
#9581=CARTESIAN_POINT('Ctrl Pts',(1.00492400591205,-0.181890537957859,0.169940289819232));
#9582=CARTESIAN_POINT('Ctrl Pts',(0.998375294985966,-0.141695629206859,
0.205111543747588));
#9583=CARTESIAN_POINT('Ctrl Pts',(0.994830026707808,-0.115492077056649,
0.221129100087819));
#9584=CARTESIAN_POINT('Ctrl Pts',(0.991238884025248,-0.0742967091364492,
0.236509675094874));
#9585=CARTESIAN_POINT('Ctrl Pts',(0.990332542620729,-0.0609922781173483,
0.24024064412003));
#9586=CARTESIAN_POINT('Ctrl Pts',(0.989696097314,-0.04763,0.242834539687907));
#9587=CARTESIAN_POINT('Origin',(0.,-0.04763,0.));
#9588=CARTESIAN_POINT('Origin',(0.,-0.04763,0.));
#9589=CARTESIAN_POINT('',(0.238183666596899,-0.04763,0.951592097314));
#9590=CARTESIAN_POINT('Origin',(0.,-0.04763,0.));
#9591=CARTESIAN_POINT('Origin',(-1.94289029309402E-16,-0.04763,1.));
#9592=CARTESIAN_POINT('Origin',(-1.94289029309402E-16,0.,1.));
#9593=CARTESIAN_POINT('',(-0.2381836665969,-0.04763,0.951592097314));
#9594=CARTESIAN_POINT('Ctrl Pts',(-0.238183666596899,-0.0476299999999999,
0.951592097314));
#9595=CARTESIAN_POINT('Ctrl Pts',(-0.233157223576062,-0.0740444353928835,
0.952850216871763));
#9596=CARTESIAN_POINT('Ctrl Pts',(-0.223801617934946,-0.0999305678883309,
0.955173119738174));
#9597=CARTESIAN_POINT('Ctrl Pts',(-0.199966927975188,-0.142345102874864,
0.960411259488514));
#9598=CARTESIAN_POINT('Ctrl Pts',(-0.1868781821531,-0.159766064500479,0.963103647174702));
#9599=CARTESIAN_POINT('Ctrl Pts',(-0.15681442133453,-0.190326085855194,
0.968453058988463));
#9600=CARTESIAN_POINT('Ctrl Pts',(-0.139836317888043,-0.203463743702801,
0.971100730005489));
#9601=CARTESIAN_POINT('Ctrl Pts',(-0.104422493053067,-0.224161999508995,
0.975530745318961));
#9602=CARTESIAN_POINT('Ctrl Pts',(-0.0842175114474176,-0.232861760990032,
0.977553872336861));
#9603=CARTESIAN_POINT('Ctrl Pts',(-0.0421062857595701,-0.244251601209411,
0.980270995488453));
#9604=CARTESIAN_POINT('Ctrl Pts',(-0.0201990724523197,-0.246942143572133,
0.980948));
#9605=CARTESIAN_POINT('Ctrl Pts',(0.020199072452319,-0.246942143572133,
0.980948));
#9606=CARTESIAN_POINT('Ctrl Pts',(0.0421062857595694,-0.244251601209411,
0.980270995488454));
#9607=CARTESIAN_POINT('Ctrl Pts',(0.0842175114474169,-0.232861760990032,
0.977553872336861));
#9608=CARTESIAN_POINT('Ctrl Pts',(0.104422493053067,-0.224161999508995,
0.975530745318961));
#9609=CARTESIAN_POINT('Ctrl Pts',(0.139836317888042,-0.203463743702801,
0.971100730005489));
#9610=CARTESIAN_POINT('Ctrl Pts',(0.15681442133453,-0.190326085855194,0.968453058988463));
#9611=CARTESIAN_POINT('Ctrl Pts',(0.1868781821531,-0.15976606450048,0.963103647174702));
#9612=CARTESIAN_POINT('Ctrl Pts',(0.199966927975188,-0.142345102874864,
0.960411259488514));
#9613=CARTESIAN_POINT('Ctrl Pts',(0.223801617934945,-0.0999305678883309,
0.955173119738174));
#9614=CARTESIAN_POINT('Ctrl Pts',(0.233157223576061,-0.0740444353928835,
0.952850216871763));
#9615=CARTESIAN_POINT('Ctrl Pts',(0.238183666596899,-0.0476299999999999,
0.951592097314));
#9616=CARTESIAN_POINT('Origin',(-1.94289029309402E-16,-0.04763,1.));
#9617=CARTESIAN_POINT('Origin',(0.,-0.04763,0.));
#9618=CARTESIAN_POINT('',(-0.504455939115715,-0.04763,0.841298510752802));
#9619=CARTESIAN_POINT('Origin',(0.,-0.04763,0.));
#9620=CARTESIAN_POINT('Origin',(-0.707106781186548,-0.04763,0.707106781186547));
#9621=CARTESIAN_POINT('Origin',(-0.707106781186548,0.,0.707106781186547));
#9622=CARTESIAN_POINT('',(-0.841298510752802,-0.04763,0.504455939115715));
#9623=CARTESIAN_POINT('Ctrl Pts',(-0.841298510752802,-0.04763,0.504455939115715));
#9624=CARTESIAN_POINT('Ctrl Pts',(-0.838633903678357,-0.0740444353928835,
0.508899795931835));
#9625=CARTESIAN_POINT('Ctrl Pts',(-0.833661031856294,-0.0999305678883309,
0.517157748491652));
#9626=CARTESIAN_POINT('Ctrl Pts',(-0.820511285096538,-0.142345102874864,
0.537715343527944));
#9627=CARTESIAN_POINT('Ctrl Pts',(-0.813159949759,-0.159766064500479,0.548874290046456));
#9628=CARTESIAN_POINT('Ctrl Pts',(-0.795684265985089,-0.190326085855194,
0.573915184558107));
#9629=CARTESIAN_POINT('Ctrl Pts',(-0.78555112003688,-0.203463743702801,
0.587792702767295));
#9630=CARTESIAN_POINT('Ctrl Pts',(-0.763642258217233,-0.224161999508995,
0.615966552324775));
#9631=CARTESIAN_POINT('Ctrl Pts',(-0.750785745543687,-0.232861760990032,
0.631684198665438));
#9632=CARTESIAN_POINT('Ctrl Pts',(-0.722929908501543,-0.244251601209411,
0.663382628119203));
#9633=CARTESIAN_POINT('Ctrl Pts',(-0.707917883896095,-0.246942143572133,
0.679352081686668));
#9634=CARTESIAN_POINT('Ctrl Pts',(-0.679352081686668,-0.246942143572133,
0.707917883896095));
#9635=CARTESIAN_POINT('Ctrl Pts',(-0.663382628119203,-0.244251601209411,
0.722929908501544));
#9636=CARTESIAN_POINT('Ctrl Pts',(-0.631684198665438,-0.232861760990031,
0.750785745543687));
#9637=CARTESIAN_POINT('Ctrl Pts',(-0.615966552324775,-0.224161999508995,
0.763642258217233));
#9638=CARTESIAN_POINT('Ctrl Pts',(-0.587792702767295,-0.203463743702801,
0.78555112003688));
#9639=CARTESIAN_POINT('Ctrl Pts',(-0.573915184558107,-0.190326085855194,
0.795684265985088));
#9640=CARTESIAN_POINT('Ctrl Pts',(-0.548874290046456,-0.159766064500479,
0.813159949759));
#9641=CARTESIAN_POINT('Ctrl Pts',(-0.537715343527944,-0.142345102874864,
0.820511285096538));
#9642=CARTESIAN_POINT('Ctrl Pts',(-0.517157748491652,-0.0999305678883309,
0.833661031856294));
#9643=CARTESIAN_POINT('Ctrl Pts',(-0.508899795931835,-0.0740444353928835,
0.838633903678357));
#9644=CARTESIAN_POINT('Ctrl Pts',(-0.504455939115716,-0.04763,0.841298510752801));
#9645=CARTESIAN_POINT('Origin',(-0.707106781186548,-0.04763,0.707106781186547));
#9646=CARTESIAN_POINT('Origin',(0.,-0.04763,0.));
#9647=CARTESIAN_POINT('',(-0.951592097314,-0.04763,0.238183666596899));
#9648=CARTESIAN_POINT('Origin',(0.,-0.04763,0.));
#9649=CARTESIAN_POINT('Origin',(-1.,-0.04763,-1.11022302462516E-16));
#9650=CARTESIAN_POINT('Origin',(-1.,0.,-1.11022302462516E-16));
#9651=CARTESIAN_POINT('',(-0.951592097314,-0.04763,-0.2381836665969));
#9652=CARTESIAN_POINT('',(-0.980948,-0.246942143572133,1.08514323328844E-18));
#9653=CARTESIAN_POINT('Ctrl Pts',(-0.951592097314,-0.04763,-0.238183666596899));
#9654=CARTESIAN_POINT('Ctrl Pts',(-0.952850216871763,-0.0740444353928835,
-0.233157223576062));
#9655=CARTESIAN_POINT('Ctrl Pts',(-0.955173119738174,-0.0999305678883309,
-0.223801617934946));
#9656=CARTESIAN_POINT('Ctrl Pts',(-0.960411259488514,-0.142345102874864,
-0.199966927975188));
#9657=CARTESIAN_POINT('Ctrl Pts',(-0.963103647174702,-0.159766064500479,
-0.1868781821531));
#9658=CARTESIAN_POINT('Ctrl Pts',(-0.968453058988463,-0.190326085855194,
-0.15681442133453));
#9659=CARTESIAN_POINT('Ctrl Pts',(-0.971100730005489,-0.203463743702801,
-0.139836317888043));
#9660=CARTESIAN_POINT('Ctrl Pts',(-0.975530745318961,-0.224161999508995,
-0.104422493053067));
#9661=CARTESIAN_POINT('Ctrl Pts',(-0.977553872336861,-0.232861760990032,
-0.0842175114474175));
#9662=CARTESIAN_POINT('Ctrl Pts',(-0.980270995488453,-0.244251601209411,
-0.0421062857595699));
#9663=CARTESIAN_POINT('Ctrl Pts',(-0.980948,-0.246942143572133,-0.0201990724523195));
#9664=CARTESIAN_POINT('Ctrl Pts',(-0.980948,-0.246942143572133,-1.17961196366423E-16));
#9665=CARTESIAN_POINT('Origin',(-1.,-0.04763,-1.11022302462516E-16));
#9666=CARTESIAN_POINT('Ctrl Pts',(-0.980948,-0.246942143572133,-1.17961196366423E-16));
#9667=CARTESIAN_POINT('Ctrl Pts',(-0.980948,-0.246942143572133,0.0201990724523192));
#9668=CARTESIAN_POINT('Ctrl Pts',(-0.980270995488453,-0.244251601209411,
0.0421062857595695));
#9669=CARTESIAN_POINT('Ctrl Pts',(-0.977553872336861,-0.232861760990032,
0.0842175114474169));
#9670=CARTESIAN_POINT('Ctrl Pts',(-0.975530745318961,-0.224161999508995,
0.104422493053066));
#9671=CARTESIAN_POINT('Ctrl Pts',(-0.971100730005489,-0.203463743702801,
0.139836317888042));
#9672=CARTESIAN_POINT('Ctrl Pts',(-0.968453058988463,-0.190326085855194,
0.15681442133453));
#9673=CARTESIAN_POINT('Ctrl Pts',(-0.963103647174702,-0.15976606450048,
0.1868781821531));
#9674=CARTESIAN_POINT('Ctrl Pts',(-0.960411259488514,-0.142345102874864,
0.199966927975188));
#9675=CARTESIAN_POINT('Ctrl Pts',(-0.955173119738174,-0.099930567888331,
0.223801617934945));
#9676=CARTESIAN_POINT('Ctrl Pts',(-0.952850216871763,-0.0740444353928835,
0.233157223576061));
#9677=CARTESIAN_POINT('Ctrl Pts',(-0.951592097314,-0.04763,0.238183666596899));
#9678=CARTESIAN_POINT('Origin',(0.,-0.04763,0.));
#9679=CARTESIAN_POINT('',(-0.841298510752802,-0.04763,-0.504455939115715));
#9680=CARTESIAN_POINT('Origin',(0.,-0.04763,0.));
#9681=CARTESIAN_POINT('Origin',(-0.707106781186547,-0.04763,-0.707106781186548));
#9682=CARTESIAN_POINT('Origin',(-0.707106781186547,0.,-0.707106781186548));
#9683=CARTESIAN_POINT('',(-0.504455939115715,-0.04763,-0.841298510752802));
#9684=CARTESIAN_POINT('Ctrl Pts',(-0.504455939115715,-0.04763,-0.841298510752802));
#9685=CARTESIAN_POINT('Ctrl Pts',(-0.508899795931835,-0.0740444353928835,
-0.838633903678357));
#9686=CARTESIAN_POINT('Ctrl Pts',(-0.517157748491652,-0.0999305678883309,
-0.833661031856294));
#9687=CARTESIAN_POINT('Ctrl Pts',(-0.537715343527944,-0.142345102874864,
-0.820511285096538));
#9688=CARTESIAN_POINT('Ctrl Pts',(-0.548874290046456,-0.159766064500479,
-0.813159949759));
#9689=CARTESIAN_POINT('Ctrl Pts',(-0.573915184558107,-0.190326085855194,
-0.795684265985089));
#9690=CARTESIAN_POINT('Ctrl Pts',(-0.587792702767295,-0.203463743702801,
-0.78555112003688));
#9691=CARTESIAN_POINT('Ctrl Pts',(-0.615966552324775,-0.224161999508995,
-0.763642258217233));
#9692=CARTESIAN_POINT('Ctrl Pts',(-0.631684198665438,-0.232861760990032,
-0.750785745543687));
#9693=CARTESIAN_POINT('Ctrl Pts',(-0.663382628119203,-0.244251601209411,
-0.722929908501543));
#9694=CARTESIAN_POINT('Ctrl Pts',(-0.679352081686668,-0.246942143572133,
-0.707917883896095));
#9695=CARTESIAN_POINT('Ctrl Pts',(-0.707917883896095,-0.246942143572133,
-0.679352081686668));
#9696=CARTESIAN_POINT('Ctrl Pts',(-0.722929908501543,-0.244251601209411,
-0.663382628119203));
#9697=CARTESIAN_POINT('Ctrl Pts',(-0.750785745543687,-0.232861760990032,
-0.631684198665439));
#9698=CARTESIAN_POINT('Ctrl Pts',(-0.763642258217232,-0.224161999508995,
-0.615966552324775));
#9699=CARTESIAN_POINT('Ctrl Pts',(-0.78555112003688,-0.203463743702801,
-0.587792702767295));
#9700=CARTESIAN_POINT('Ctrl Pts',(-0.795684265985088,-0.190326085855194,
-0.573915184558107));
#9701=CARTESIAN_POINT('Ctrl Pts',(-0.813159949759,-0.15976606450048,-0.548874290046456));
#9702=CARTESIAN_POINT('Ctrl Pts',(-0.820511285096538,-0.142345102874864,
-0.537715343527944));
#9703=CARTESIAN_POINT('Ctrl Pts',(-0.833661031856294,-0.0999305678883311,
-0.517157748491652));
#9704=CARTESIAN_POINT('Ctrl Pts',(-0.838633903678357,-0.0740444353928836,
-0.508899795931835));
#9705=CARTESIAN_POINT('Ctrl Pts',(-0.841298510752801,-0.04763,-0.504455939115715));
#9706=CARTESIAN_POINT('Origin',(-0.707106781186547,-0.04763,-0.707106781186548));
#9707=CARTESIAN_POINT('Origin',(0.,-0.04763,0.));
#9708=CARTESIAN_POINT('',(-0.238183666596899,-0.04763,-0.951592097314));
#9709=CARTESIAN_POINT('Origin',(0.,-0.04763,0.));
#9710=CARTESIAN_POINT('Origin',(5.55111512312578E-17,-0.04763,-1.));
#9711=CARTESIAN_POINT('Origin',(5.55111512312578E-17,0.,-1.));
#9712=CARTESIAN_POINT('',(0.238183666596899,-0.04763,-0.951592097314));
#9713=CARTESIAN_POINT('Ctrl Pts',(0.238183666596899,-0.04763,-0.951592097314));
#9714=CARTESIAN_POINT('Ctrl Pts',(0.233157223576062,-0.0740444353928835,
-0.952850216871763));
#9715=CARTESIAN_POINT('Ctrl Pts',(0.223801617934946,-0.099930567888331,
-0.955173119738174));
#9716=CARTESIAN_POINT('Ctrl Pts',(0.199966927975188,-0.142345102874864,
-0.960411259488514));
#9717=CARTESIAN_POINT('Ctrl Pts',(0.1868781821531,-0.15976606450048,-0.963103647174702));
#9718=CARTESIAN_POINT('Ctrl Pts',(0.15681442133453,-0.190326085855194,-0.968453058988463));
#9719=CARTESIAN_POINT('Ctrl Pts',(0.139836317888042,-0.203463743702801,
-0.971100730005489));
#9720=CARTESIAN_POINT('Ctrl Pts',(0.104422493053067,-0.224161999508995,
-0.975530745318961));
#9721=CARTESIAN_POINT('Ctrl Pts',(0.0842175114474173,-0.232861760990032,
-0.977553872336861));
#9722=CARTESIAN_POINT('Ctrl Pts',(0.0421062857595698,-0.244251601209411,
-0.980270995488453));
#9723=CARTESIAN_POINT('Ctrl Pts',(0.0201990724523194,-0.246942143572133,
-0.980948));
#9724=CARTESIAN_POINT('Ctrl Pts',(-0.0201990724523193,-0.246942143572133,
-0.980948));
#9725=CARTESIAN_POINT('Ctrl Pts',(-0.0421062857595697,-0.244251601209411,
-0.980270995488453));
#9726=CARTESIAN_POINT('Ctrl Pts',(-0.0842175114474171,-0.232861760990032,
-0.977553872336861));
#9727=CARTESIAN_POINT('Ctrl Pts',(-0.104422493053067,-0.224161999508995,
-0.975530745318961));
#9728=CARTESIAN_POINT('Ctrl Pts',(-0.139836317888042,-0.203463743702801,
-0.971100730005489));
#9729=CARTESIAN_POINT('Ctrl Pts',(-0.15681442133453,-0.190326085855194,
-0.968453058988463));
#9730=CARTESIAN_POINT('Ctrl Pts',(-0.1868781821531,-0.15976606450048,-0.963103647174702));
#9731=CARTESIAN_POINT('Ctrl Pts',(-0.199966927975188,-0.142345102874864,
-0.960411259488514));
#9732=CARTESIAN_POINT('Ctrl Pts',(-0.223801617934945,-0.099930567888331,
-0.955173119738174));
#9733=CARTESIAN_POINT('Ctrl Pts',(-0.233157223576062,-0.0740444353928835,
-0.952850216871763));
#9734=CARTESIAN_POINT('Ctrl Pts',(-0.238183666596899,-0.0476299999999999,
-0.951592097314));
#9735=CARTESIAN_POINT('Origin',(5.55111512312578E-17,-0.04763,-1.));
#9736=CARTESIAN_POINT('Origin',(0.,-0.04763,0.));
#9737=CARTESIAN_POINT('',(0.504455939115715,-0.04763,-0.841298510752802));
#9738=CARTESIAN_POINT('Origin',(0.,-0.04763,0.));
#9739=CARTESIAN_POINT('Origin',(0.707106781186548,-0.04763,-0.707106781186547));
#9740=CARTESIAN_POINT('Origin',(0.707106781186548,0.,-0.707106781186547));
#9741=CARTESIAN_POINT('',(0.841298510752802,-0.04763,-0.504455939115715));
#9742=CARTESIAN_POINT('Ctrl Pts',(0.841298510752802,-0.04763,-0.504455939115715));
#9743=CARTESIAN_POINT('Ctrl Pts',(0.838633903678357,-0.0740444353928835,
-0.508899795931835));
#9744=CARTESIAN_POINT('Ctrl Pts',(0.833661031856294,-0.0999305678883309,
-0.517157748491652));
#9745=CARTESIAN_POINT('Ctrl Pts',(0.820511285096538,-0.142345102874864,
-0.537715343527944));
#9746=CARTESIAN_POINT('Ctrl Pts',(0.813159949759,-0.159766064500479,-0.548874290046456));
#9747=CARTESIAN_POINT('Ctrl Pts',(0.795684265985088,-0.190326085855194,
-0.573915184558107));
#9748=CARTESIAN_POINT('Ctrl Pts',(0.78555112003688,-0.203463743702801,-0.587792702767295));
#9749=CARTESIAN_POINT('Ctrl Pts',(0.763642258217233,-0.224161999508995,
-0.615966552324775));
#9750=CARTESIAN_POINT('Ctrl Pts',(0.750785745543687,-0.232861760990032,
-0.631684198665438));
#9751=CARTESIAN_POINT('Ctrl Pts',(0.722929908501543,-0.244251601209411,
-0.663382628119203));
#9752=CARTESIAN_POINT('Ctrl Pts',(0.707917883896095,-0.246942143572133,
-0.679352081686668));
#9753=CARTESIAN_POINT('Ctrl Pts',(0.679352081686668,-0.246942143572133,
-0.707917883896095));
#9754=CARTESIAN_POINT('Ctrl Pts',(0.663382628119203,-0.244251601209411,
-0.722929908501543));
#9755=CARTESIAN_POINT('Ctrl Pts',(0.631684198665438,-0.232861760990032,
-0.750785745543687));
#9756=CARTESIAN_POINT('Ctrl Pts',(0.615966552324775,-0.224161999508995,
-0.763642258217232));
#9757=CARTESIAN_POINT('Ctrl Pts',(0.587792702767295,-0.203463743702801,
-0.78555112003688));
#9758=CARTESIAN_POINT('Ctrl Pts',(0.573915184558107,-0.190326085855194,
-0.795684265985088));
#9759=CARTESIAN_POINT('Ctrl Pts',(0.548874290046456,-0.159766064500479,
-0.813159949759));
#9760=CARTESIAN_POINT('Ctrl Pts',(0.537715343527944,-0.142345102874864,
-0.820511285096538));
#9761=CARTESIAN_POINT('Ctrl Pts',(0.517157748491652,-0.099930567888331,
-0.833661031856294));
#9762=CARTESIAN_POINT('Ctrl Pts',(0.508899795931835,-0.0740444353928835,
-0.838633903678357));
#9763=CARTESIAN_POINT('Ctrl Pts',(0.504455939115715,-0.04763,-0.841298510752801));
#9764=CARTESIAN_POINT('Origin',(0.707106781186548,-0.04763,-0.707106781186547));
#9765=CARTESIAN_POINT('Origin',(0.,-0.166705,0.));
#9766=CARTESIAN_POINT('',(-0.980948,-0.28578,1.20131482833E-16));
#9767=CARTESIAN_POINT('Origin',(0.,-0.28578,0.));
#9768=CARTESIAN_POINT('',(-0.980948,-0.166705,1.20131482833E-16));
#9769=CARTESIAN_POINT('',(0.951592097314,-0.04763,0.238183666596899));
#9770=CARTESIAN_POINT('Origin',(0.,-0.04763,0.));
#9771=CARTESIAN_POINT('',(0.951592097314,-0.04763,-0.238183666596899));
#9772=CARTESIAN_POINT('Ctrl Pts',(0.951592097314,-0.04763,0.238183666596899));
#9773=CARTESIAN_POINT('Ctrl Pts',(0.952850216871763,-0.0740444353928835,
0.233157223576062));
#9774=CARTESIAN_POINT('Ctrl Pts',(0.955173119738174,-0.099930567888331,
0.223801617934945));
#9775=CARTESIAN_POINT('Ctrl Pts',(0.960411259488514,-0.142345102874864,
0.199966927975188));
#9776=CARTESIAN_POINT('Ctrl Pts',(0.963103647174702,-0.15976606450048,0.1868781821531));
#9777=CARTESIAN_POINT('Ctrl Pts',(0.968453058988463,-0.190326085855194,
0.15681442133453));
#9778=CARTESIAN_POINT('Ctrl Pts',(0.971100730005489,-0.203463743702801,
0.139836317888042));
#9779=CARTESIAN_POINT('Ctrl Pts',(0.975530745318961,-0.224161999508995,
0.104422493053067));
#9780=CARTESIAN_POINT('Ctrl Pts',(0.977553872336861,-0.232861760990032,
0.0842175114474172));
#9781=CARTESIAN_POINT('Ctrl Pts',(0.980270995488453,-0.244251601209411,
0.0421062857595697));
#9782=CARTESIAN_POINT('Ctrl Pts',(0.980948,-0.246942143572133,0.0201990724523194));
#9783=CARTESIAN_POINT('Ctrl Pts',(0.980948,-0.246942143572133,-0.0201990724523194));
#9784=CARTESIAN_POINT('Ctrl Pts',(0.980270995488453,-0.244251601209411,
-0.0421062857595697));
#9785=CARTESIAN_POINT('Ctrl Pts',(0.977553872336861,-0.232861760990032,
-0.0842175114474172));
#9786=CARTESIAN_POINT('Ctrl Pts',(0.975530745318961,-0.224161999508995,
-0.104422493053067));
#9787=CARTESIAN_POINT('Ctrl Pts',(0.971100730005489,-0.203463743702801,
-0.139836317888042));
#9788=CARTESIAN_POINT('Ctrl Pts',(0.968453058988463,-0.190326085855194,
-0.15681442133453));
#9789=CARTESIAN_POINT('Ctrl Pts',(0.963103647174702,-0.15976606450048,-0.1868781821531));
#9790=CARTESIAN_POINT('Ctrl Pts',(0.960411259488514,-0.142345102874864,
-0.199966927975188));
#9791=CARTESIAN_POINT('Ctrl Pts',(0.955173119738174,-0.099930567888331,
-0.223801617934945));
#9792=CARTESIAN_POINT('Ctrl Pts',(0.952850216871763,-0.0740444353928835,
-0.233157223576062));
#9793=CARTESIAN_POINT('Ctrl Pts',(0.951592097314,-0.0476299999999999,-0.238183666596899));
#9794=CARTESIAN_POINT('Origin',(0.,-0.04763,0.));
#9795=CARTESIAN_POINT('Origin',(0.,-0.04763,0.));
#9796=CARTESIAN_POINT('Origin',(1.,-0.04763,0.));
#9797=CARTESIAN_POINT('Origin',(1.,0.,0.));
#9798=CARTESIAN_POINT('Origin',(1.,-0.04763,0.));
#9799=CARTESIAN_POINT('Origin',(0.,-0.28578,0.));
#9800=CARTESIAN_POINT('Origin',(0.,-0.04763,0.));
#10909=UNCERTAINTY_MEASURE_WITH_UNIT(LENGTH_MEASURE(0.001),#10958,
'DISTANCE_ACCURACY_VALUE',
'Maximum model space distance between geometric entities at asserted c
onnectivities');
#10926=UNCERTAINTY_MEASURE_WITH_UNIT(LENGTH_MEASURE(0.001),#10958,
'DISTANCE_ACCURACY_VALUE',
'Maximum model space distance between geometric entities at asserted c
onnectivities');
#10940=(
GEOMETRIC_REPRESENTATION_CONTEXT(3)
GLOBAL_UNCERTAINTY_ASSIGNED_CONTEXT((#10909))
GLOBAL_UNIT_ASSIGNED_CONTEXT((#10958,#10960,#10961))
REPRESENTATION_CONTEXT('','3D')
);
#10957=(
GEOMETRIC_REPRESENTATION_CONTEXT(3)
GLOBAL_UNCERTAINTY_ASSIGNED_CONTEXT((#10926))
GLOBAL_UNIT_ASSIGNED_CONTEXT((#10958,#10960,#10961))
REPRESENTATION_CONTEXT('','3D')
);
#10958=(
LENGTH_UNIT()
NAMED_UNIT(*)
SI_UNIT(.CENTI.,.METRE.)
);
#10960=(
NAMED_UNIT(*)
PLANE_ANGLE_UNIT()
SI_UNIT($,.RADIAN.)
);
#10961=(
NAMED_UNIT(*)
SI_UNIT($,.STERADIAN.)
SOLID_ANGLE_UNIT()
);
#10975=SHAPE_DEFINITION_REPRESENTATION(#11005,#11077);
#11005=PRODUCT_DEFINITION_SHAPE('',$,#11108);
#11077=SHAPE_REPRESENTATION('',(#6328),#10940);
#11094=PRODUCT_DEFINITION_CONTEXT('part definition',#11186,'design');
#11108=PRODUCT_DEFINITION('Cage','Cage',#11138,#11094);
#11138=PRODUCT_DEFINITION_FORMATION('',$,#11201);
#11186=APPLICATION_CONTEXT(
'Core Data for Automotive Mechanical Design Process');
#11187=PRODUCT_CONTEXT('part definition',#11186,'mechanical');
#11201=PRODUCT('Cage','Cage','Cage',(#11187));
#11281=COLOUR_RGB('Grey',0.48,0.52,0.57);
#11282=FILL_AREA_STYLE_COLOUR('',#11281);
#11283=FILL_AREA_STYLE('',(#11282));
#11284=SURFACE_STYLE_FILL_AREA(#11283);
#11285=SURFACE_SIDE_STYLE('',(#11284));
#11286=SURFACE_STYLE_USAGE(.BOTH.,#11285);
#11287=PRESENTATION_STYLE_ASSIGNMENT((#11286));
ENDSEC;
END-ISO-10303-21;
